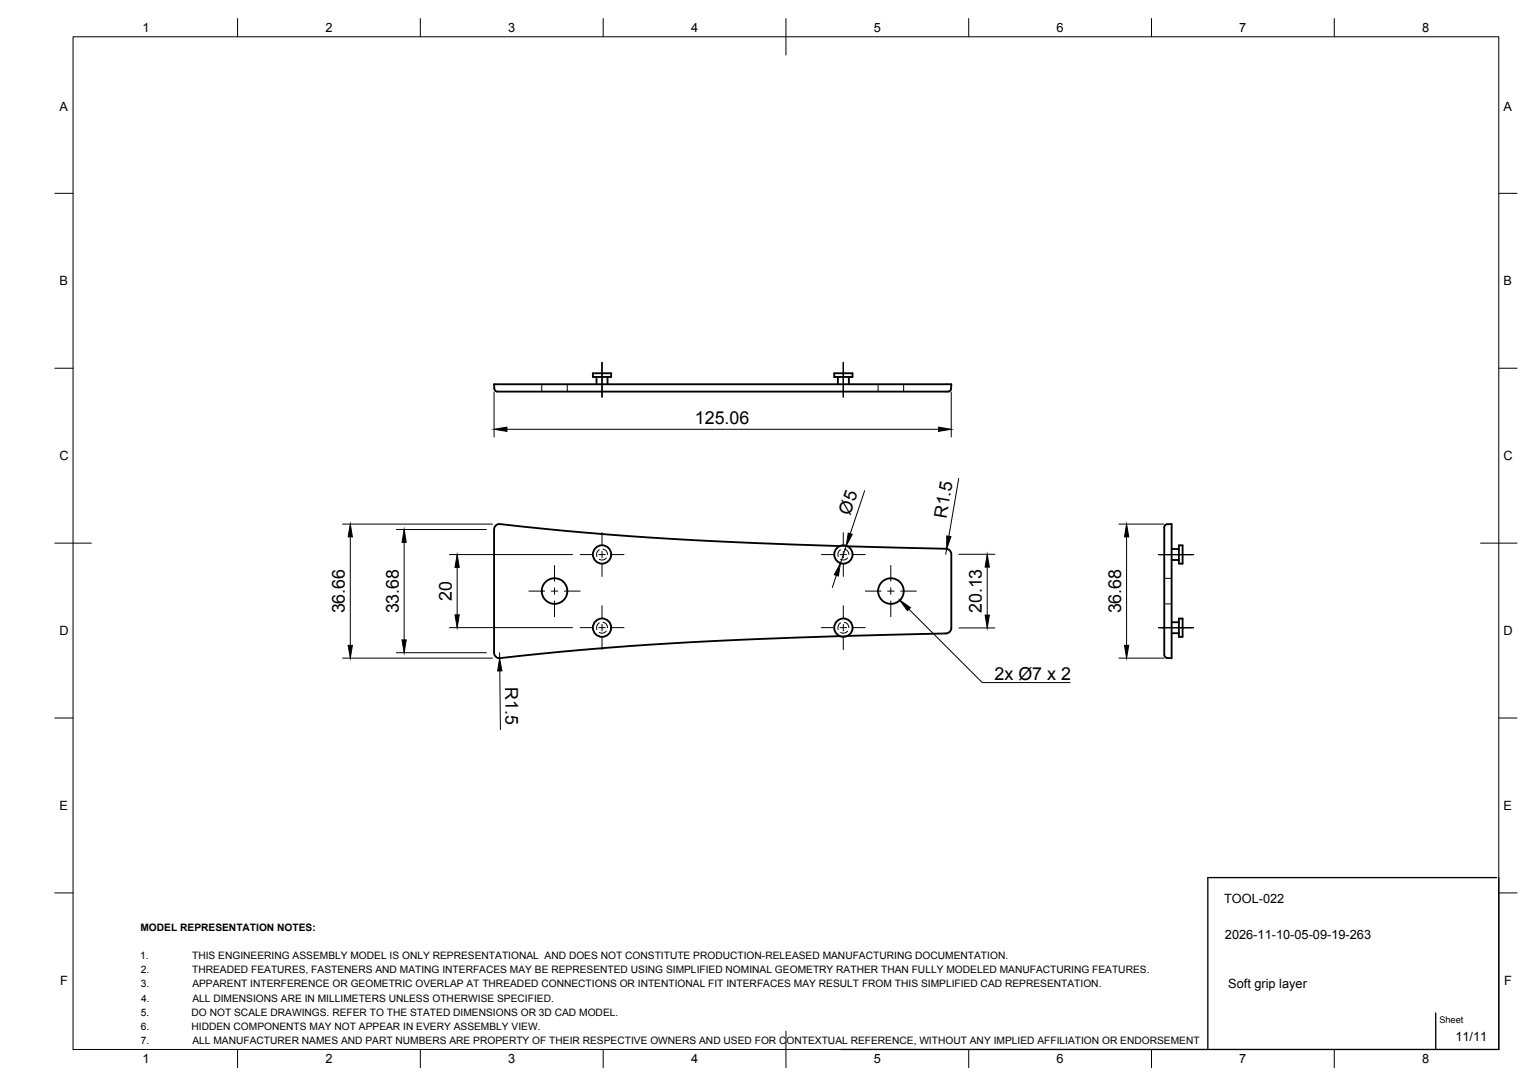
ISO-10303-21;
HEADER;
/* Generated by software containing ST-Developer
 * from STEP Tools, Inc. (www.steptools.com) 
 */

FILE_DESCRIPTION(
/* description */ (''),
/* implementation_level */ '2;1');

FILE_NAME(
/* name */ 'Soft grip layer.step',
/* time_stamp */ '2026-11-10T08:27:36-08:00',
/* author */ (''),
/* organization */ (''),
/* preprocessor_version */ 'ST-DEVELOPER v20.2',
/* originating_system */ 'Autodesk Translation Framework v15.17.0.0',
/* authorisation */ '');

FILE_SCHEMA (('AUTOMOTIVE_DESIGN { 1 0 10303 214 3 1 1 }'));
ENDSEC;

DATA;
#10=MECHANICAL_DESIGN_GEOMETRIC_PRESENTATION_REPRESENTATION('',(#572),#19090);
#156=B_SPLINE_SURFACE_WITH_KNOTS('',3,3,((#13418,#13419,#13420,#13421,#13422),
(#13423,#13424,#13425,#13426,#13427),(#13428,#13429,#13430,#13431,#13432),
(#13433,#13434,#13435,#13436,#13437),(#13438,#13439,#13440,#13441,#13442)),
 .UNSPECIFIED.,.F.,.F.,.F.,(4,1,4),(4,1,4),(0.,0.571428571428571,1.),(0.,
0.0505788685273923,0.118017359897249),.UNSPECIFIED.);
#157=B_SPLINE_SURFACE_WITH_KNOTS('',3,3,((#13465,#13466,#13467,#13468,#13469),
(#13470,#13471,#13472,#13473,#13474),(#13475,#13476,#13477,#13478,#13479),
(#13480,#13481,#13482,#13483,#13484),(#13485,#13486,#13487,#13488,#13489)),
 .UNSPECIFIED.,.F.,.F.,.F.,(4,1,4),(4,1,4),(0.,0.571428571428571,1.),(0.,
0.0505788685278266,0.118017359898262),.UNSPECIFIED.);
#158=B_SPLINE_SURFACE_WITH_KNOTS('',3,3,((#13503,#13504,#13505,#13506,#13507),
(#13508,#13509,#13510,#13511,#13512),(#13513,#13514,#13515,#13516,#13517),
(#13518,#13519,#13520,#13521,#13522),(#13523,#13524,#13525,#13526,#13527)),
 .UNSPECIFIED.,.F.,.F.,.F.,(4,1,4),(4,1,4),(0.,0.571428571428571,1.),(0.,
5.23288834931112,12.2100728150593),.UNSPECIFIED.);
#159=B_SPLINE_SURFACE_WITH_KNOTS('',3,3,((#13541,#13542,#13543,#13544,#13545),
(#13546,#13547,#13548,#13549,#13550),(#13551,#13552,#13553,#13554,#13555),
(#13556,#13557,#13558,#13559,#13560),(#13561,#13562,#13563,#13564,#13565)),
 .UNSPECIFIED.,.F.,.F.,.F.,(4,1,4),(4,1,4),(0.,0.571428571428571,1.),(1.97133828064127E-11,
0.0463413823988794,0.108129892237767),.UNSPECIFIED.);
#160=B_SPLINE_SURFACE_WITH_KNOTS('',3,3,((#13585,#13586,#13587,#13588,#13589),
(#13590,#13591,#13592,#13593,#13594),(#13595,#13596,#13597,#13598,#13599),
(#13600,#13601,#13602,#13603,#13604),(#13605,#13606,#13607,#13608,#13609)),
 .UNSPECIFIED.,.F.,.F.,.F.,(4,1,4),(4,1,4),(0.,0.571428571428571,1.),(0.,
0.0463413823743492,0.108129892206815),.UNSPECIFIED.);
#161=B_SPLINE_SURFACE_WITH_KNOTS('',3,3,((#13623,#13624,#13625,#13626,#13627),
(#13628,#13629,#13630,#13631,#13632),(#13633,#13634,#13635,#13636,#13637),
(#13638,#13639,#13640,#13641,#13642),(#13643,#13644,#13645,#13646,#13647)),
 .UNSPECIFIED.,.F.,.F.,.F.,(4,1,4),(4,1,4),(0.,0.571428571428571,1.),(6.51086303075479E-13,
6.97718480957529,12.2100734167563),.UNSPECIFIED.);
#162=B_SPLINE_SURFACE_WITH_KNOTS('',3,3,((#13670,#13671,#13672,#13673),
(#13674,#13675,#13676,#13677),(#13678,#13679,#13680,#13681),(#13682,#13683,
#13684,#13685),(#13686,#13687,#13688,#13689)),.UNSPECIFIED.,.F.,.F.,.F.,
(4,1,4),(4,4),(0.,0.571428571428571,1.),(-0.00308447593286339,0.124708996845866),
 .UNSPECIFIED.);
#163=B_SPLINE_SURFACE_WITH_KNOTS('',3,3,((#13723,#13724,#13725,#13726),
(#13727,#13728,#13729,#13730),(#13731,#13732,#13733,#13734),(#13735,#13736,
#13737,#13738)),.UNSPECIFIED.,.F.,.F.,.F.,(4,4),(4,4),(0.0116899650356219,
0.986620910196183),(0.,0.621418053543664),.UNSPECIFIED.);
#164=B_SPLINE_SURFACE_WITH_KNOTS('',3,3,((#13748,#13749,#13750,#13751),
(#13752,#13753,#13754,#13755),(#13756,#13757,#13758,#13759),(#13760,#13761,
#13762,#13763),(#13764,#13765,#13766,#13767),(#13768,#13769,#13770,#13771)),
 .UNSPECIFIED.,.F.,.F.,.F.,(4,1,1,4),(4,4),(0.,0.285714285714286,0.571428571428571,
1.),(-0.00421817271916687,0.124025126494243),.UNSPECIFIED.);
#165=B_SPLINE_SURFACE_WITH_KNOTS('',3,3,((#13819,#13820,#13821,#13822),
(#13823,#13824,#13825,#13826),(#13827,#13828,#13829,#13830),(#13831,#13832,
#13833,#13834),(#13835,#13836,#13837,#13838)),.UNSPECIFIED.,.F.,.F.,.F.,
(4,1,4),(4,4),(0.,0.571428571428571,1.),(-0.00306862226109154,0.124708996851356),
 .UNSPECIFIED.);
#166=B_SPLINE_SURFACE_WITH_KNOTS('',3,3,((#13872,#13873,#13874,#13875),
(#13876,#13877,#13878,#13879),(#13880,#13881,#13882,#13883),(#13884,#13885,
#13886,#13887),(#13888,#13889,#13890,#13891),(#13892,#13893,#13894,#13895)),
 .UNSPECIFIED.,.F.,.F.,.F.,(4,1,1,4),(4,4),(0.,0.285714285714286,0.571428571428571,
1.),(-0.00430078538920315,0.12402512649425),.UNSPECIFIED.);
#167=B_SPLINE_SURFACE_WITH_KNOTS('',3,3,((#13940,#13941,#13942,#13943),
(#13944,#13945,#13946,#13947),(#13948,#13949,#13950,#13951),(#13952,#13953,
#13954,#13955)),.UNSPECIFIED.,.F.,.F.,.F.,(4,4),(4,4),(0.0133790898038168,
0.988310034964378),(0.,0.621418053491537),.UNSPECIFIED.);
#364=B_SPLINE_CURVE_WITH_KNOTS('',3,(#13447,#13448,#13449,#13450,#13451),
 .UNSPECIFIED.,.F.,.F.,(4,1,4),(-0.118017359897249,-0.0505788685273923,
0.),.UNSPECIFIED.);
#365=B_SPLINE_CURVE_WITH_KNOTS('',3,(#13454,#13455,#13456,#13457,#13458),
 .UNSPECIFIED.,.F.,.F.,(4,1,4),(0.,0.0505788685273923,0.118017359897249),
 .UNSPECIFIED.);
#366=B_SPLINE_CURVE_WITH_KNOTS('',3,(#13493,#13494,#13495,#13496,#13497),
 .UNSPECIFIED.,.F.,.F.,(4,1,4),(-0.118017359898262,-0.0505788685278266,
0.),.UNSPECIFIED.);
#367=B_SPLINE_CURVE_WITH_KNOTS('',3,(#13498,#13499,#13500,#13501,#13502),
 .UNSPECIFIED.,.F.,.F.,(4,1,4),(0.,0.0505788685278266,0.118017359898262),
 .UNSPECIFIED.);
#368=B_SPLINE_CURVE_WITH_KNOTS('',3,(#13531,#13532,#13533,#13534,#13535),
 .UNSPECIFIED.,.F.,.F.,(4,1,4),(-12.2100728150593,-5.23288834931112,0.),
 .UNSPECIFIED.);
#369=B_SPLINE_CURVE_WITH_KNOTS('',3,(#13536,#13537,#13538,#13539,#13540),
 .UNSPECIFIED.,.F.,.F.,(4,1,4),(0.,5.23288834931112,12.2100728150593),
 .UNSPECIFIED.);
#370=B_SPLINE_CURVE_WITH_KNOTS('',3,(#13569,#13570,#13571,#13572,#13573),
 .UNSPECIFIED.,.F.,.F.,(4,1,4),(-0.108129892237767,-0.0463413823988794,
-1.97133828064127E-11),.UNSPECIFIED.);
#371=B_SPLINE_CURVE_WITH_KNOTS('',3,(#13574,#13575,#13576,#13577,#13578),
 .UNSPECIFIED.,.F.,.F.,(4,1,4),(1.97133828064127E-11,0.0463413823988794,
0.108129892237767),.UNSPECIFIED.);
#372=B_SPLINE_CURVE_WITH_KNOTS('',3,(#13613,#13614,#13615,#13616,#13617),
 .UNSPECIFIED.,.F.,.F.,(4,1,4),(-0.108129892206815,-0.0463413823743492,
0.),.UNSPECIFIED.);
#373=B_SPLINE_CURVE_WITH_KNOTS('',3,(#13618,#13619,#13620,#13621,#13622),
 .UNSPECIFIED.,.F.,.F.,(4,1,4),(0.,0.0463413823743492,0.108129892206815),
 .UNSPECIFIED.);
#374=B_SPLINE_CURVE_WITH_KNOTS('',3,(#13648,#13649,#13650,#13651,#13652),
 .UNSPECIFIED.,.F.,.F.,(4,1,4),(-12.2100734167563,-6.97718480957529,-6.51086303075479E-13),
 .UNSPECIFIED.);
#375=B_SPLINE_CURVE_WITH_KNOTS('',3,(#13653,#13654,#13655,#13656,#13657),
 .UNSPECIFIED.,.F.,.F.,(4,1,4),(6.51086303075479E-13,6.97718480957529,12.2100734167563),
 .UNSPECIFIED.);
#376=B_SPLINE_CURVE_WITH_KNOTS('',3,(#13660,#13661,#13662,#13663),
 .UNSPECIFIED.,.F.,.F.,(4,4),(0.000181689894813921,0.124708996845866),
 .UNSPECIFIED.);
#377=B_SPLINE_CURVE_WITH_KNOTS('',3,(#13666,#13667,#13668,#13669),
 .UNSPECIFIED.,.F.,.F.,(4,4),(-0.124708996851356,-0.000181689894814102),
 .UNSPECIFIED.);
#378=B_SPLINE_CURVE_WITH_KNOTS('',3,(#13691,#13692,#13693,#13694),
 .UNSPECIFIED.,.F.,.F.,(4,4),(-0.124624122980966,-1.27068494615301E-16),
 .UNSPECIFIED.);
#379=B_SPLINE_CURVE_WITH_KNOTS('',3,(#13695,#13696,#13697,#13698,#13699,
#13700,#13701,#13702,#13703,#13704,#13705,#13706,#13707,#13708,#13709,#13710,
#13711,#13712,#13713,#13714,#13715,#13716,#13717,#13718,#13719,#13720,#13721,
#13722),.UNSPECIFIED.,.F.,.F.,(4,3,3,3,3,3,3,3,3,4),(0.,0.0322747504276753,
0.0586406101183928,0.090870813631105,0.0996503787243826,0.117132790114159,
0.149546322800321,0.175583390425035,0.207787925145658,0.232457773984835),
 .UNSPECIFIED.);
#380=B_SPLINE_CURVE_WITH_KNOTS('',3,(#13740,#13741,#13742,#13743),
 .UNSPECIFIED.,.F.,.F.,(4,4),(6.28713621962651E-9,0.124025126494243),
 .UNSPECIFIED.);
#381=B_SPLINE_CURVE_WITH_KNOTS('',3,(#13744,#13745,#13746,#13747),
 .UNSPECIFIED.,.F.,.F.,(4,4),(0.0116899650356219,0.986620910196183),
 .UNSPECIFIED.);
#382=B_SPLINE_CURVE_WITH_KNOTS('',3,(#13773,#13774,#13775,#13776),
 .UNSPECIFIED.,.F.,.F.,(4,4),(-0.12358375933533,0.000944809985246663),
 .UNSPECIFIED.);
#383=B_SPLINE_CURVE_WITH_KNOTS('',3,(#13777,#13778,#13779,#13780,#13781,
#13782,#13783,#13784,#13785,#13786,#13787,#13788,#13789,#13790,#13791,#13792,
#13793,#13794,#13795,#13796,#13797,#13798,#13799,#13800,#13801,#13802,#13803,
#13804,#13805,#13806,#13807,#13808,#13809,#13810),.UNSPECIFIED.,.F.,.F.,
(4,3,3,3,3,3,3,3,3,3,3,4),(0.,0.0322568536241053,0.0586526138523664,0.0909514856947606,
0.108742407475907,0.117151788463556,0.149394351344039,0.175600627102286,
0.181167420983902,0.214570374458228,0.246736309066329,0.253563811229603),
 .UNSPECIFIED.);
#384=B_SPLINE_CURVE_WITH_KNOTS('',3,(#13814,#13815,#13816,#13817),
 .UNSPECIFIED.,.F.,.F.,(4,4),(-0.000944809985246617,0.123583759335329),
 .UNSPECIFIED.);
#385=B_SPLINE_CURVE_WITH_KNOTS('',3,(#13840,#13841,#13842,#13843,#13844,
#13845,#13846,#13847,#13848,#13849,#13850,#13851,#13852,#13853,#13854,#13855,
#13856,#13857,#13858,#13859,#13860,#13861,#13862,#13863,#13864,#13865,#13866,
#13867),.UNSPECIFIED.,.F.,.F.,(4,3,3,3,3,3,3,3,3,4),(0.,0.0322765438584903,
0.0586513922310012,0.0908809480268686,0.099655003871439,0.117150238497558,
0.149564657711791,0.175599638586681,0.20780211537115,0.232458396023953),
 .UNSPECIFIED.);
#386=B_SPLINE_CURVE_WITH_KNOTS('',3,(#13868,#13869,#13870,#13871),
 .UNSPECIFIED.,.F.,.F.,(4,4),(3.30031141304588E-16,0.124624122970512),
 .UNSPECIFIED.);
#387=B_SPLINE_CURVE_WITH_KNOTS('',3,(#13897,#13898,#13899,#13900),
 .UNSPECIFIED.,.F.,.F.,(4,4),(-0.12402512649425,-6.28713634712869E-9),
 .UNSPECIFIED.);
#388=B_SPLINE_CURVE_WITH_KNOTS('',3,(#13901,#13902,#13903,#13904,#13905,
#13906,#13907,#13908,#13909,#13910,#13911,#13912,#13913,#13914,#13915,#13916,
#13917,#13918,#13919,#13920,#13921,#13922,#13923,#13924,#13925,#13926,#13927,
#13928,#13929,#13930,#13931,#13932,#13933,#13934),.UNSPECIFIED.,.F.,.F.,
(4,3,3,3,3,3,3,3,3,3,3,4),(0.,0.0322666769662355,0.0587055335553437,0.0910029078093924,
0.108768157423115,0.117242626226166,0.149488313345073,0.175692943342501,
0.181189289804584,0.214619150478997,0.24677571115805,0.253566775541772),
 .UNSPECIFIED.);
#389=B_SPLINE_CURVE_WITH_KNOTS('',3,(#13936,#13937,#13938,#13939),
 .UNSPECIFIED.,.F.,.F.,(4,4),(0.0133790898038168,0.988310034964378),
 .UNSPECIFIED.);
#552=SHAPE_REPRESENTATION_RELATIONSHIP('SRR','None',#19143,#562);
#562=ADVANCED_BREP_SHAPE_REPRESENTATION('',(#582),#19086);
#572=STYLED_ITEM('',(#19204),#582);
#582=MANIFOLD_SOLID_BREP('Body1',#6826);
#635=FACE_BOUND('',#1503,.T.);
#636=FACE_BOUND('',#1507,.T.);
#637=FACE_BOUND('',#1511,.T.);
#638=FACE_BOUND('',#1515,.T.);
#639=FACE_BOUND('',#1535,.T.);
#640=FACE_BOUND('',#1536,.T.);
#641=FACE_BOUND('',#1541,.T.);
#642=FACE_BOUND('',#1542,.T.);
#643=FACE_BOUND('',#1543,.T.);
#644=FACE_BOUND('',#1544,.T.);
#645=FACE_BOUND('',#1545,.T.);
#646=FACE_BOUND('',#1546,.T.);
#781=PLANE('',#7258);
#782=PLANE('',#7263);
#783=PLANE('',#7264);
#784=PLANE('',#7269);
#785=PLANE('',#7270);
#786=PLANE('',#7275);
#787=PLANE('',#7276);
#788=PLANE('',#7281);
#789=PLANE('',#7300);
#790=PLANE('',#7301);
#791=PLANE('',#7302);
#792=PLANE('',#7303);
#1063=FACE_OUTER_BOUND('',#1500,.T.);
#1064=FACE_OUTER_BOUND('',#1501,.T.);
#1065=FACE_OUTER_BOUND('',#1502,.T.);
#1066=FACE_OUTER_BOUND('',#1504,.T.);
#1067=FACE_OUTER_BOUND('',#1505,.T.);
#1068=FACE_OUTER_BOUND('',#1506,.T.);
#1069=FACE_OUTER_BOUND('',#1508,.T.);
#1070=FACE_OUTER_BOUND('',#1509,.T.);
#1071=FACE_OUTER_BOUND('',#1510,.T.);
#1072=FACE_OUTER_BOUND('',#1512,.T.);
#1073=FACE_OUTER_BOUND('',#1513,.T.);
#1074=FACE_OUTER_BOUND('',#1514,.T.);
#1075=FACE_OUTER_BOUND('',#1516,.T.);
#1076=FACE_OUTER_BOUND('',#1517,.T.);
#1077=FACE_OUTER_BOUND('',#1518,.T.);
#1078=FACE_OUTER_BOUND('',#1519,.T.);
#1079=FACE_OUTER_BOUND('',#1520,.T.);
#1080=FACE_OUTER_BOUND('',#1521,.T.);
#1081=FACE_OUTER_BOUND('',#1522,.T.);
#1082=FACE_OUTER_BOUND('',#1523,.T.);
#1083=FACE_OUTER_BOUND('',#1524,.T.);
#1084=FACE_OUTER_BOUND('',#1525,.T.);
#1085=FACE_OUTER_BOUND('',#1526,.T.);
#1086=FACE_OUTER_BOUND('',#1527,.T.);
#1087=FACE_OUTER_BOUND('',#1528,.T.);
#1088=FACE_OUTER_BOUND('',#1529,.T.);
#1089=FACE_OUTER_BOUND('',#1530,.T.);
#1090=FACE_OUTER_BOUND('',#1531,.T.);
#1091=FACE_OUTER_BOUND('',#1532,.T.);
#1092=FACE_OUTER_BOUND('',#1533,.T.);
#1093=FACE_OUTER_BOUND('',#1534,.T.);
#1094=FACE_OUTER_BOUND('',#1537,.T.);
#1095=FACE_OUTER_BOUND('',#1538,.T.);
#1096=FACE_OUTER_BOUND('',#1539,.T.);
#1097=FACE_OUTER_BOUND('',#1540,.T.);
#1098=FACE_OUTER_BOUND('',#1547,.T.);
#1500=EDGE_LOOP('',(#5597,#5598,#5599,#5600));
#1501=EDGE_LOOP('',(#5601,#5602,#5603,#5604));
#1502=EDGE_LOOP('',(#5605));
#1503=EDGE_LOOP('',(#5606));
#1504=EDGE_LOOP('',(#5607,#5608,#5609,#5610));
#1505=EDGE_LOOP('',(#5611));
#1506=EDGE_LOOP('',(#5612));
#1507=EDGE_LOOP('',(#5613));
#1508=EDGE_LOOP('',(#5614,#5615,#5616,#5617));
#1509=EDGE_LOOP('',(#5618));
#1510=EDGE_LOOP('',(#5619));
#1511=EDGE_LOOP('',(#5620));
#1512=EDGE_LOOP('',(#5621,#5622,#5623,#5624));
#1513=EDGE_LOOP('',(#5625));
#1514=EDGE_LOOP('',(#5626));
#1515=EDGE_LOOP('',(#5627));
#1516=EDGE_LOOP('',(#5628,#5629,#5630,#5631));
#1517=EDGE_LOOP('',(#5632));
#1518=EDGE_LOOP('',(#5633,#5634,#5635,#5636));
#1519=EDGE_LOOP('',(#5637,#5638,#5639,#5640));
#1520=EDGE_LOOP('',(#5641,#5642,#5643,#5644));
#1521=EDGE_LOOP('',(#5645,#5646,#5647,#5648));
#1522=EDGE_LOOP('',(#5649,#5650,#5651,#5652));
#1523=EDGE_LOOP('',(#5653,#5654,#5655,#5656));
#1524=EDGE_LOOP('',(#5657,#5658,#5659,#5660));
#1525=EDGE_LOOP('',(#5661,#5662,#5663,#5664));
#1526=EDGE_LOOP('',(#5665,#5666,#5667,#5668));
#1527=EDGE_LOOP('',(#5669,#5670,#5671,#5672));
#1528=EDGE_LOOP('',(#5673,#5674,#5675,#5676));
#1529=EDGE_LOOP('',(#5677,#5678,#5679,#5680));
#1530=EDGE_LOOP('',(#5681,#5682,#5683,#5684));
#1531=EDGE_LOOP('',(#5685,#5686,#5687,#5688));
#1532=EDGE_LOOP('',(#5689,#5690,#5691,#5692));
#1533=EDGE_LOOP('',(#5693,#5694,#5695,#5696));
#1534=EDGE_LOOP('',(#5697,#5698,#5699,#5700,#5701,#5702,#5703,#5704));
#1535=EDGE_LOOP('',(#5705));
#1536=EDGE_LOOP('',(#5706));
#1537=EDGE_LOOP('',(#5707,#5708,#5709,#5710));
#1538=EDGE_LOOP('',(#5711,#5712,#5713,#5714));
#1539=EDGE_LOOP('',(#5715,#5716,#5717,#5718));
#1540=EDGE_LOOP('',(#5719,#5720,#5721,#5722,#5723,#5724,#5725,#5726));
#1541=EDGE_LOOP('',(#5727));
#1542=EDGE_LOOP('',(#5728));
#1543=EDGE_LOOP('',(#5729));
#1544=EDGE_LOOP('',(#5730));
#1545=EDGE_LOOP('',(#5731));
#1546=EDGE_LOOP('',(#5732));
#1547=EDGE_LOOP('',(#5733,#5734,#5735,#5736));
#1979=LINE('',#13354,#2428);
#1980=LINE('',#13360,#2429);
#1981=LINE('',#13370,#2430);
#1982=LINE('',#13380,#2431);
#1983=LINE('',#13390,#2432);
#1984=LINE('',#13400,#2433);
#1985=LINE('',#13404,#2434);
#1986=LINE('',#13408,#2435);
#1987=LINE('',#13412,#2436);
#1988=LINE('',#13416,#2437);
#1989=LINE('',#13463,#2438);
#1990=LINE('',#13464,#2439);
#1991=LINE('',#13583,#2440);
#1992=LINE('',#13584,#2441);
#1993=LINE('',#13665,#2442);
#1994=LINE('',#13818,#2443);
#2428=VECTOR('',#8386,0.35);
#2429=VECTOR('',#8393,0.35);
#2430=VECTOR('',#8406,0.25);
#2431=VECTOR('',#8419,0.25);
#2432=VECTOR('',#8432,0.25);
#2433=VECTOR('',#8445,0.25);
#2434=VECTOR('',#8450,0.15);
#2435=VECTOR('',#8455,0.15);
#2436=VECTOR('',#8460,0.15);
#2437=VECTOR('',#8465,0.15);
#2438=VECTOR('',#8476,1.);
#2439=VECTOR('',#8477,1.);
#2440=VECTOR('',#8488,1.);
#2441=VECTOR('',#8489,1.);
#2442=VECTOR('',#8494,1.);
#2443=VECTOR('',#8499,1.);
#2670=CIRCLE('',#7253,0.35);
#2671=CIRCLE('',#7254,0.35);
#2672=CIRCLE('',#7256,0.35);
#2673=CIRCLE('',#7257,0.35);
#2674=CIRCLE('',#7259,0.25);
#2675=CIRCLE('',#7260,0.15);
#2676=CIRCLE('',#7262,0.25);
#2677=CIRCLE('',#7265,0.25);
#2678=CIRCLE('',#7266,0.15);
#2679=CIRCLE('',#7268,0.25);
#2680=CIRCLE('',#7271,0.25);
#2681=CIRCLE('',#7272,0.15);
#2682=CIRCLE('',#7274,0.25);
#2683=CIRCLE('',#7277,0.25);
#2684=CIRCLE('',#7278,0.15);
#2685=CIRCLE('',#7280,0.25);
#2686=CIRCLE('',#7283,0.15);
#2687=CIRCLE('',#7285,0.15);
#2688=CIRCLE('',#7287,0.15);
#2689=CIRCLE('',#7289,0.15);
#2690=CIRCLE('',#7290,0.0800000000000001);
#2691=CIRCLE('',#7291,0.0800000000000001);
#2692=CIRCLE('',#7293,0.0800000000000001);
#2693=CIRCLE('',#7294,0.0800000000000001);
#2694=CIRCLE('',#7295,0.0800000000000001);
#2695=CIRCLE('',#7296,0.0800000000000003);
#2696=CIRCLE('',#7298,0.0800000000000001);
#2697=CIRCLE('',#7299,0.0800000000000003);
#3120=VERTEX_POINT('',#13351);
#3121=VERTEX_POINT('',#13353);
#3122=VERTEX_POINT('',#13357);
#3123=VERTEX_POINT('',#13359);
#3124=VERTEX_POINT('',#13363);
#3125=VERTEX_POINT('',#13365);
#3126=VERTEX_POINT('',#13368);
#3127=VERTEX_POINT('',#13373);
#3128=VERTEX_POINT('',#13375);
#3129=VERTEX_POINT('',#13378);
#3130=VERTEX_POINT('',#13383);
#3131=VERTEX_POINT('',#13385);
#3132=VERTEX_POINT('',#13388);
#3133=VERTEX_POINT('',#13393);
#3134=VERTEX_POINT('',#13395);
#3135=VERTEX_POINT('',#13398);
#3136=VERTEX_POINT('',#13403);
#3137=VERTEX_POINT('',#13407);
#3138=VERTEX_POINT('',#13411);
#3139=VERTEX_POINT('',#13415);
#3140=VERTEX_POINT('',#13443);
#3141=VERTEX_POINT('',#13444);
#3142=VERTEX_POINT('',#13446);
#3143=VERTEX_POINT('',#13452);
#3144=VERTEX_POINT('',#13460);
#3145=VERTEX_POINT('',#13461);
#3146=VERTEX_POINT('',#13490);
#3147=VERTEX_POINT('',#13491);
#3148=VERTEX_POINT('',#13528);
#3149=VERTEX_POINT('',#13529);
#3150=VERTEX_POINT('',#13566);
#3151=VERTEX_POINT('',#13567);
#3152=VERTEX_POINT('',#13580);
#3153=VERTEX_POINT('',#13581);
#3154=VERTEX_POINT('',#13610);
#3155=VERTEX_POINT('',#13611);
#3156=VERTEX_POINT('',#13659);
#3157=VERTEX_POINT('',#13664);
#3158=VERTEX_POINT('',#13690);
#3159=VERTEX_POINT('',#13739);
#3160=VERTEX_POINT('',#13772);
#3161=VERTEX_POINT('',#13813);
#3162=VERTEX_POINT('',#13839);
#3163=VERTEX_POINT('',#13896);
#3983=EDGE_CURVE('',#3120,#3120,#2670,.T.);
#3984=EDGE_CURVE('',#3120,#3121,#1979,.T.);
#3985=EDGE_CURVE('',#3121,#3121,#2671,.T.);
#3986=EDGE_CURVE('',#3122,#3122,#2672,.T.);
#3987=EDGE_CURVE('',#3122,#3123,#1980,.T.);
#3988=EDGE_CURVE('',#3123,#3123,#2673,.T.);
#3989=EDGE_CURVE('',#3124,#3124,#2674,.T.);
#3990=EDGE_CURVE('',#3125,#3125,#2675,.T.);
#3991=EDGE_CURVE('',#3126,#3126,#2676,.T.);
#3992=EDGE_CURVE('',#3126,#3124,#1981,.T.);
#3993=EDGE_CURVE('',#3127,#3127,#2677,.T.);
#3994=EDGE_CURVE('',#3128,#3128,#2678,.T.);
#3995=EDGE_CURVE('',#3129,#3129,#2679,.T.);
#3996=EDGE_CURVE('',#3129,#3127,#1982,.T.);
#3997=EDGE_CURVE('',#3130,#3130,#2680,.T.);
#3998=EDGE_CURVE('',#3131,#3131,#2681,.T.);
#3999=EDGE_CURVE('',#3132,#3132,#2682,.T.);
#4000=EDGE_CURVE('',#3132,#3130,#1983,.T.);
#4001=EDGE_CURVE('',#3133,#3133,#2683,.T.);
#4002=EDGE_CURVE('',#3134,#3134,#2684,.T.);
#4003=EDGE_CURVE('',#3135,#3135,#2685,.T.);
#4004=EDGE_CURVE('',#3135,#3133,#1984,.T.);
#4005=EDGE_CURVE('',#3125,#3136,#1985,.T.);
#4006=EDGE_CURVE('',#3136,#3136,#2686,.T.);
#4007=EDGE_CURVE('',#3128,#3137,#1986,.T.);
#4008=EDGE_CURVE('',#3137,#3137,#2687,.T.);
#4009=EDGE_CURVE('',#3131,#3138,#1987,.T.);
#4010=EDGE_CURVE('',#3138,#3138,#2688,.T.);
#4011=EDGE_CURVE('',#3134,#3139,#1988,.T.);
#4012=EDGE_CURVE('',#3139,#3139,#2689,.T.);
#4013=EDGE_CURVE('',#3140,#3141,#2690,.T.);
#4014=EDGE_CURVE('',#3141,#3142,#364,.T.);
#4015=EDGE_CURVE('',#3142,#3143,#2691,.T.);
#4016=EDGE_CURVE('',#3143,#3140,#365,.T.);
#4017=EDGE_CURVE('',#3144,#3145,#2692,.T.);
#4018=EDGE_CURVE('',#3145,#3141,#1989,.T.);
#4019=EDGE_CURVE('',#3140,#3144,#1990,.T.);
#4020=EDGE_CURVE('',#3146,#3147,#2693,.T.);
#4021=EDGE_CURVE('',#3147,#3145,#366,.T.);
#4022=EDGE_CURVE('',#3144,#3146,#367,.T.);
#4023=EDGE_CURVE('',#3148,#3149,#2694,.T.);
#4024=EDGE_CURVE('',#3149,#3147,#368,.T.);
#4025=EDGE_CURVE('',#3146,#3148,#369,.T.);
#4026=EDGE_CURVE('',#3150,#3151,#2695,.T.);
#4027=EDGE_CURVE('',#3151,#3149,#370,.T.);
#4028=EDGE_CURVE('',#3148,#3150,#371,.T.);
#4029=EDGE_CURVE('',#3152,#3153,#2696,.T.);
#4030=EDGE_CURVE('',#3153,#3151,#1991,.T.);
#4031=EDGE_CURVE('',#3150,#3152,#1992,.T.);
#4032=EDGE_CURVE('',#3154,#3155,#2697,.T.);
#4033=EDGE_CURVE('',#3155,#3153,#372,.T.);
#4034=EDGE_CURVE('',#3152,#3154,#373,.T.);
#4035=EDGE_CURVE('',#3142,#3155,#374,.T.);
#4036=EDGE_CURVE('',#3154,#3143,#375,.T.);
#4037=EDGE_CURVE('',#3156,#3153,#376,.T.);
#4038=EDGE_CURVE('',#3157,#3156,#1993,.T.);
#4039=EDGE_CURVE('',#3151,#3157,#377,.T.);
#4040=EDGE_CURVE('',#3155,#3158,#378,.T.);
#4041=EDGE_CURVE('',#3158,#3156,#379,.T.);
#4042=EDGE_CURVE('',#3159,#3142,#380,.T.);
#4043=EDGE_CURVE('',#3158,#3159,#381,.T.);
#4044=EDGE_CURVE('',#3141,#3160,#382,.T.);
#4045=EDGE_CURVE('',#3160,#3159,#383,.T.);
#4046=EDGE_CURVE('',#3161,#3145,#384,.T.);
#4047=EDGE_CURVE('',#3160,#3161,#1994,.T.);
#4048=EDGE_CURVE('',#3157,#3162,#385,.T.);
#4049=EDGE_CURVE('',#3162,#3149,#386,.T.);
#4050=EDGE_CURVE('',#3147,#3163,#387,.T.);
#4051=EDGE_CURVE('',#3163,#3161,#388,.T.);
#4052=EDGE_CURVE('',#3163,#3162,#389,.T.);
#5597=ORIENTED_EDGE('',*,*,#3983,.F.);
#5598=ORIENTED_EDGE('',*,*,#3984,.T.);
#5599=ORIENTED_EDGE('',*,*,#3985,.F.);
#5600=ORIENTED_EDGE('',*,*,#3984,.F.);
#5601=ORIENTED_EDGE('',*,*,#3986,.F.);
#5602=ORIENTED_EDGE('',*,*,#3987,.T.);
#5603=ORIENTED_EDGE('',*,*,#3988,.F.);
#5604=ORIENTED_EDGE('',*,*,#3987,.F.);
#5605=ORIENTED_EDGE('',*,*,#3989,.T.);
#5606=ORIENTED_EDGE('',*,*,#3990,.T.);
#5607=ORIENTED_EDGE('',*,*,#3991,.F.);
#5608=ORIENTED_EDGE('',*,*,#3992,.T.);
#5609=ORIENTED_EDGE('',*,*,#3989,.F.);
#5610=ORIENTED_EDGE('',*,*,#3992,.F.);
#5611=ORIENTED_EDGE('',*,*,#3991,.T.);
#5612=ORIENTED_EDGE('',*,*,#3993,.T.);
#5613=ORIENTED_EDGE('',*,*,#3994,.T.);
#5614=ORIENTED_EDGE('',*,*,#3995,.F.);
#5615=ORIENTED_EDGE('',*,*,#3996,.T.);
#5616=ORIENTED_EDGE('',*,*,#3993,.F.);
#5617=ORIENTED_EDGE('',*,*,#3996,.F.);
#5618=ORIENTED_EDGE('',*,*,#3995,.T.);
#5619=ORIENTED_EDGE('',*,*,#3997,.T.);
#5620=ORIENTED_EDGE('',*,*,#3998,.T.);
#5621=ORIENTED_EDGE('',*,*,#3999,.F.);
#5622=ORIENTED_EDGE('',*,*,#4000,.T.);
#5623=ORIENTED_EDGE('',*,*,#3997,.F.);
#5624=ORIENTED_EDGE('',*,*,#4000,.F.);
#5625=ORIENTED_EDGE('',*,*,#3999,.T.);
#5626=ORIENTED_EDGE('',*,*,#4001,.T.);
#5627=ORIENTED_EDGE('',*,*,#4002,.T.);
#5628=ORIENTED_EDGE('',*,*,#4003,.F.);
#5629=ORIENTED_EDGE('',*,*,#4004,.T.);
#5630=ORIENTED_EDGE('',*,*,#4001,.F.);
#5631=ORIENTED_EDGE('',*,*,#4004,.F.);
#5632=ORIENTED_EDGE('',*,*,#4003,.T.);
#5633=ORIENTED_EDGE('',*,*,#3990,.F.);
#5634=ORIENTED_EDGE('',*,*,#4005,.T.);
#5635=ORIENTED_EDGE('',*,*,#4006,.F.);
#5636=ORIENTED_EDGE('',*,*,#4005,.F.);
#5637=ORIENTED_EDGE('',*,*,#3994,.F.);
#5638=ORIENTED_EDGE('',*,*,#4007,.T.);
#5639=ORIENTED_EDGE('',*,*,#4008,.F.);
#5640=ORIENTED_EDGE('',*,*,#4007,.F.);
#5641=ORIENTED_EDGE('',*,*,#3998,.F.);
#5642=ORIENTED_EDGE('',*,*,#4009,.T.);
#5643=ORIENTED_EDGE('',*,*,#4010,.F.);
#5644=ORIENTED_EDGE('',*,*,#4009,.F.);
#5645=ORIENTED_EDGE('',*,*,#4002,.F.);
#5646=ORIENTED_EDGE('',*,*,#4011,.T.);
#5647=ORIENTED_EDGE('',*,*,#4012,.F.);
#5648=ORIENTED_EDGE('',*,*,#4011,.F.);
#5649=ORIENTED_EDGE('',*,*,#4013,.T.);
#5650=ORIENTED_EDGE('',*,*,#4014,.T.);
#5651=ORIENTED_EDGE('',*,*,#4015,.T.);
#5652=ORIENTED_EDGE('',*,*,#4016,.T.);
#5653=ORIENTED_EDGE('',*,*,#4017,.T.);
#5654=ORIENTED_EDGE('',*,*,#4018,.T.);
#5655=ORIENTED_EDGE('',*,*,#4013,.F.);
#5656=ORIENTED_EDGE('',*,*,#4019,.T.);
#5657=ORIENTED_EDGE('',*,*,#4020,.T.);
#5658=ORIENTED_EDGE('',*,*,#4021,.T.);
#5659=ORIENTED_EDGE('',*,*,#4017,.F.);
#5660=ORIENTED_EDGE('',*,*,#4022,.T.);
#5661=ORIENTED_EDGE('',*,*,#4023,.T.);
#5662=ORIENTED_EDGE('',*,*,#4024,.T.);
#5663=ORIENTED_EDGE('',*,*,#4020,.F.);
#5664=ORIENTED_EDGE('',*,*,#4025,.T.);
#5665=ORIENTED_EDGE('',*,*,#4026,.T.);
#5666=ORIENTED_EDGE('',*,*,#4027,.T.);
#5667=ORIENTED_EDGE('',*,*,#4023,.F.);
#5668=ORIENTED_EDGE('',*,*,#4028,.T.);
#5669=ORIENTED_EDGE('',*,*,#4029,.T.);
#5670=ORIENTED_EDGE('',*,*,#4030,.T.);
#5671=ORIENTED_EDGE('',*,*,#4026,.F.);
#5672=ORIENTED_EDGE('',*,*,#4031,.T.);
#5673=ORIENTED_EDGE('',*,*,#4032,.T.);
#5674=ORIENTED_EDGE('',*,*,#4033,.T.);
#5675=ORIENTED_EDGE('',*,*,#4029,.F.);
#5676=ORIENTED_EDGE('',*,*,#4034,.T.);
#5677=ORIENTED_EDGE('',*,*,#4015,.F.);
#5678=ORIENTED_EDGE('',*,*,#4035,.T.);
#5679=ORIENTED_EDGE('',*,*,#4032,.F.);
#5680=ORIENTED_EDGE('',*,*,#4036,.T.);
#5681=ORIENTED_EDGE('',*,*,#4030,.F.);
#5682=ORIENTED_EDGE('',*,*,#4037,.F.);
#5683=ORIENTED_EDGE('',*,*,#4038,.F.);
#5684=ORIENTED_EDGE('',*,*,#4039,.F.);
#5685=ORIENTED_EDGE('',*,*,#4033,.F.);
#5686=ORIENTED_EDGE('',*,*,#4040,.T.);
#5687=ORIENTED_EDGE('',*,*,#4041,.T.);
#5688=ORIENTED_EDGE('',*,*,#4037,.T.);
#5689=ORIENTED_EDGE('',*,*,#4035,.F.);
#5690=ORIENTED_EDGE('',*,*,#4042,.F.);
#5691=ORIENTED_EDGE('',*,*,#4043,.F.);
#5692=ORIENTED_EDGE('',*,*,#4040,.F.);
#5693=ORIENTED_EDGE('',*,*,#4014,.F.);
#5694=ORIENTED_EDGE('',*,*,#4044,.T.);
#5695=ORIENTED_EDGE('',*,*,#4045,.T.);
#5696=ORIENTED_EDGE('',*,*,#4042,.T.);
#5697=ORIENTED_EDGE('',*,*,#4016,.F.);
#5698=ORIENTED_EDGE('',*,*,#4036,.F.);
#5699=ORIENTED_EDGE('',*,*,#4034,.F.);
#5700=ORIENTED_EDGE('',*,*,#4031,.F.);
#5701=ORIENTED_EDGE('',*,*,#4028,.F.);
#5702=ORIENTED_EDGE('',*,*,#4025,.F.);
#5703=ORIENTED_EDGE('',*,*,#4022,.F.);
#5704=ORIENTED_EDGE('',*,*,#4019,.F.);
#5705=ORIENTED_EDGE('',*,*,#3983,.T.);
#5706=ORIENTED_EDGE('',*,*,#3986,.T.);
#5707=ORIENTED_EDGE('',*,*,#4018,.F.);
#5708=ORIENTED_EDGE('',*,*,#4046,.F.);
#5709=ORIENTED_EDGE('',*,*,#4047,.F.);
#5710=ORIENTED_EDGE('',*,*,#4044,.F.);
#5711=ORIENTED_EDGE('',*,*,#4027,.F.);
#5712=ORIENTED_EDGE('',*,*,#4039,.T.);
#5713=ORIENTED_EDGE('',*,*,#4048,.T.);
#5714=ORIENTED_EDGE('',*,*,#4049,.T.);
#5715=ORIENTED_EDGE('',*,*,#4021,.F.);
#5716=ORIENTED_EDGE('',*,*,#4050,.T.);
#5717=ORIENTED_EDGE('',*,*,#4051,.T.);
#5718=ORIENTED_EDGE('',*,*,#4046,.T.);
#5719=ORIENTED_EDGE('',*,*,#4045,.F.);
#5720=ORIENTED_EDGE('',*,*,#4047,.T.);
#5721=ORIENTED_EDGE('',*,*,#4051,.F.);
#5722=ORIENTED_EDGE('',*,*,#4052,.T.);
#5723=ORIENTED_EDGE('',*,*,#4048,.F.);
#5724=ORIENTED_EDGE('',*,*,#4038,.T.);
#5725=ORIENTED_EDGE('',*,*,#4041,.F.);
#5726=ORIENTED_EDGE('',*,*,#4043,.T.);
#5727=ORIENTED_EDGE('',*,*,#3985,.T.);
#5728=ORIENTED_EDGE('',*,*,#3988,.T.);
#5729=ORIENTED_EDGE('',*,*,#4006,.T.);
#5730=ORIENTED_EDGE('',*,*,#4008,.T.);
#5731=ORIENTED_EDGE('',*,*,#4010,.T.);
#5732=ORIENTED_EDGE('',*,*,#4012,.T.);
#5733=ORIENTED_EDGE('',*,*,#4024,.F.);
#5734=ORIENTED_EDGE('',*,*,#4049,.F.);
#5735=ORIENTED_EDGE('',*,*,#4052,.F.);
#5736=ORIENTED_EDGE('',*,*,#4050,.F.);
#6343=CYLINDRICAL_SURFACE('',#7252,0.35);
#6344=CYLINDRICAL_SURFACE('',#7255,0.35);
#6345=CYLINDRICAL_SURFACE('',#7261,0.25);
#6346=CYLINDRICAL_SURFACE('',#7267,0.25);
#6347=CYLINDRICAL_SURFACE('',#7273,0.25);
#6348=CYLINDRICAL_SURFACE('',#7279,0.25);
#6349=CYLINDRICAL_SURFACE('',#7282,0.15);
#6350=CYLINDRICAL_SURFACE('',#7284,0.15);
#6351=CYLINDRICAL_SURFACE('',#7286,0.15);
#6352=CYLINDRICAL_SURFACE('',#7288,0.15);
#6353=CYLINDRICAL_SURFACE('',#7292,0.08);
#6354=CYLINDRICAL_SURFACE('',#7297,0.08);
#6682=ADVANCED_FACE('',(#1063),#6343,.F.);
#6683=ADVANCED_FACE('',(#1064),#6344,.F.);
#6684=ADVANCED_FACE('',(#1065,#635),#781,.T.);
#6685=ADVANCED_FACE('',(#1066),#6345,.T.);
#6686=ADVANCED_FACE('',(#1067),#782,.F.);
#6687=ADVANCED_FACE('',(#1068,#636),#783,.T.);
#6688=ADVANCED_FACE('',(#1069),#6346,.T.);
#6689=ADVANCED_FACE('',(#1070),#784,.F.);
#6690=ADVANCED_FACE('',(#1071,#637),#785,.T.);
#6691=ADVANCED_FACE('',(#1072),#6347,.T.);
#6692=ADVANCED_FACE('',(#1073),#786,.F.);
#6693=ADVANCED_FACE('',(#1074,#638),#787,.T.);
#6694=ADVANCED_FACE('',(#1075),#6348,.T.);
#6695=ADVANCED_FACE('',(#1076),#788,.F.);
#6696=ADVANCED_FACE('',(#1077),#6349,.T.);
#6697=ADVANCED_FACE('',(#1078),#6350,.T.);
#6698=ADVANCED_FACE('',(#1079),#6351,.T.);
#6699=ADVANCED_FACE('',(#1080),#6352,.T.);
#6700=ADVANCED_FACE('',(#1081),#156,.F.);
#6701=ADVANCED_FACE('',(#1082),#6353,.T.);
#6702=ADVANCED_FACE('',(#1083),#157,.F.);
#6703=ADVANCED_FACE('',(#1084),#158,.F.);
#6704=ADVANCED_FACE('',(#1085),#159,.F.);
#6705=ADVANCED_FACE('',(#1086),#6354,.T.);
#6706=ADVANCED_FACE('',(#1087),#160,.F.);
#6707=ADVANCED_FACE('',(#1088),#161,.F.);
#6708=ADVANCED_FACE('',(#1089),#789,.F.);
#6709=ADVANCED_FACE('',(#1090),#162,.F.);
#6710=ADVANCED_FACE('',(#1091),#163,.F.);
#6711=ADVANCED_FACE('',(#1092),#164,.F.);
#6712=ADVANCED_FACE('',(#1093,#639,#640),#790,.T.);
#6713=ADVANCED_FACE('',(#1094),#791,.F.);
#6714=ADVANCED_FACE('',(#1095),#165,.F.);
#6715=ADVANCED_FACE('',(#1096),#166,.F.);
#6716=ADVANCED_FACE('',(#1097,#641,#642,#643,#644,#645,#646),#792,.F.);
#6717=ADVANCED_FACE('',(#1098),#167,.F.);
#6826=CLOSED_SHELL('',(#6682,#6683,#6684,#6685,#6686,#6687,#6688,#6689,
#6690,#6691,#6692,#6693,#6694,#6695,#6696,#6697,#6698,#6699,#6700,#6701,
#6702,#6703,#6704,#6705,#6706,#6707,#6708,#6709,#6710,#6711,#6712,#6713,
#6714,#6715,#6716,#6717));
#7251=AXIS2_PLACEMENT_3D('',#13349,#8380,#8381);
#7252=AXIS2_PLACEMENT_3D('',#13350,#8382,#8383);
#7253=AXIS2_PLACEMENT_3D('',#13352,#8384,#8385);
#7254=AXIS2_PLACEMENT_3D('',#13355,#8387,#8388);
#7255=AXIS2_PLACEMENT_3D('',#13356,#8389,#8390);
#7256=AXIS2_PLACEMENT_3D('',#13358,#8391,#8392);
#7257=AXIS2_PLACEMENT_3D('',#13361,#8394,#8395);
#7258=AXIS2_PLACEMENT_3D('',#13362,#8396,#8397);
#7259=AXIS2_PLACEMENT_3D('',#13364,#8398,#8399);
#7260=AXIS2_PLACEMENT_3D('',#13366,#8400,#8401);
#7261=AXIS2_PLACEMENT_3D('',#13367,#8402,#8403);
#7262=AXIS2_PLACEMENT_3D('',#13369,#8404,#8405);
#7263=AXIS2_PLACEMENT_3D('',#13371,#8407,#8408);
#7264=AXIS2_PLACEMENT_3D('',#13372,#8409,#8410);
#7265=AXIS2_PLACEMENT_3D('',#13374,#8411,#8412);
#7266=AXIS2_PLACEMENT_3D('',#13376,#8413,#8414);
#7267=AXIS2_PLACEMENT_3D('',#13377,#8415,#8416);
#7268=AXIS2_PLACEMENT_3D('',#13379,#8417,#8418);
#7269=AXIS2_PLACEMENT_3D('',#13381,#8420,#8421);
#7270=AXIS2_PLACEMENT_3D('',#13382,#8422,#8423);
#7271=AXIS2_PLACEMENT_3D('',#13384,#8424,#8425);
#7272=AXIS2_PLACEMENT_3D('',#13386,#8426,#8427);
#7273=AXIS2_PLACEMENT_3D('',#13387,#8428,#8429);
#7274=AXIS2_PLACEMENT_3D('',#13389,#8430,#8431);
#7275=AXIS2_PLACEMENT_3D('',#13391,#8433,#8434);
#7276=AXIS2_PLACEMENT_3D('',#13392,#8435,#8436);
#7277=AXIS2_PLACEMENT_3D('',#13394,#8437,#8438);
#7278=AXIS2_PLACEMENT_3D('',#13396,#8439,#8440);
#7279=AXIS2_PLACEMENT_3D('',#13397,#8441,#8442);
#7280=AXIS2_PLACEMENT_3D('',#13399,#8443,#8444);
#7281=AXIS2_PLACEMENT_3D('',#13401,#8446,#8447);
#7282=AXIS2_PLACEMENT_3D('',#13402,#8448,#8449);
#7283=AXIS2_PLACEMENT_3D('',#13405,#8451,#8452);
#7284=AXIS2_PLACEMENT_3D('',#13406,#8453,#8454);
#7285=AXIS2_PLACEMENT_3D('',#13409,#8456,#8457);
#7286=AXIS2_PLACEMENT_3D('',#13410,#8458,#8459);
#7287=AXIS2_PLACEMENT_3D('',#13413,#8461,#8462);
#7288=AXIS2_PLACEMENT_3D('',#13414,#8463,#8464);
#7289=AXIS2_PLACEMENT_3D('',#13417,#8466,#8467);
#7290=AXIS2_PLACEMENT_3D('',#13445,#8468,#8469);
#7291=AXIS2_PLACEMENT_3D('',#13453,#8470,#8471);
#7292=AXIS2_PLACEMENT_3D('',#13459,#8472,#8473);
#7293=AXIS2_PLACEMENT_3D('',#13462,#8474,#8475);
#7294=AXIS2_PLACEMENT_3D('',#13492,#8478,#8479);
#7295=AXIS2_PLACEMENT_3D('',#13530,#8480,#8481);
#7296=AXIS2_PLACEMENT_3D('',#13568,#8482,#8483);
#7297=AXIS2_PLACEMENT_3D('',#13579,#8484,#8485);
#7298=AXIS2_PLACEMENT_3D('',#13582,#8486,#8487);
#7299=AXIS2_PLACEMENT_3D('',#13612,#8490,#8491);
#7300=AXIS2_PLACEMENT_3D('',#13658,#8492,#8493);
#7301=AXIS2_PLACEMENT_3D('',#13811,#8495,#8496);
#7302=AXIS2_PLACEMENT_3D('',#13812,#8497,#8498);
#7303=AXIS2_PLACEMENT_3D('',#13935,#8500,#8501);
#8380=DIRECTION('axis',(0.,0.,1.));
#8381=DIRECTION('refdir',(1.,0.,0.));
#8382=DIRECTION('center_axis',(0.,0.,-1.));
#8383=DIRECTION('ref_axis',(1.,0.,0.));
#8384=DIRECTION('center_axis',(-6.04309184969008E-32,-6.38489691472444E-32,
-1.));
#8385=DIRECTION('ref_axis',(1.,0.,0.));
#8386=DIRECTION('',(0.,0.,-1.));
#8387=DIRECTION('center_axis',(1.44549646912992E-31,1.50240180416177E-18,
1.));
#8388=DIRECTION('ref_axis',(1.,0.,0.));
#8389=DIRECTION('center_axis',(0.,0.,-1.));
#8390=DIRECTION('ref_axis',(1.,0.,0.));
#8391=DIRECTION('center_axis',(-6.04309184969008E-32,-6.38489691472444E-32,
-1.));
#8392=DIRECTION('ref_axis',(1.,0.,0.));
#8393=DIRECTION('',(0.,0.,-1.));
#8394=DIRECTION('center_axis',(1.44549646912992E-31,1.50240180416177E-18,
1.));
#8395=DIRECTION('ref_axis',(1.,0.,0.));
#8396=DIRECTION('center_axis',(0.,0.,1.));
#8397=DIRECTION('ref_axis',(1.,0.,0.));
#8398=DIRECTION('center_axis',(0.,0.,1.));
#8399=DIRECTION('ref_axis',(1.,0.,0.));
#8400=DIRECTION('center_axis',(0.,0.,-1.));
#8401=DIRECTION('ref_axis',(1.,0.,0.));
#8402=DIRECTION('center_axis',(0.,0.,-1.));
#8403=DIRECTION('ref_axis',(1.,0.,0.));
#8404=DIRECTION('center_axis',(0.,0.,-1.));
#8405=DIRECTION('ref_axis',(1.,0.,0.));
#8406=DIRECTION('',(0.,0.,1.));
#8407=DIRECTION('center_axis',(0.,0.,1.));
#8408=DIRECTION('ref_axis',(1.,0.,0.));
#8409=DIRECTION('center_axis',(0.,0.,1.));
#8410=DIRECTION('ref_axis',(1.,0.,0.));
#8411=DIRECTION('center_axis',(0.,0.,1.));
#8412=DIRECTION('ref_axis',(1.,0.,0.));
#8413=DIRECTION('center_axis',(0.,0.,-1.));
#8414=DIRECTION('ref_axis',(1.,0.,0.));
#8415=DIRECTION('center_axis',(0.,0.,-1.));
#8416=DIRECTION('ref_axis',(1.,0.,0.));
#8417=DIRECTION('center_axis',(0.,0.,-1.));
#8418=DIRECTION('ref_axis',(1.,0.,0.));
#8419=DIRECTION('',(0.,0.,1.));
#8420=DIRECTION('center_axis',(0.,0.,1.));
#8421=DIRECTION('ref_axis',(1.,0.,0.));
#8422=DIRECTION('center_axis',(0.,0.,1.));
#8423=DIRECTION('ref_axis',(1.,0.,0.));
#8424=DIRECTION('center_axis',(0.,0.,1.));
#8425=DIRECTION('ref_axis',(1.,0.,0.));
#8426=DIRECTION('center_axis',(0.,0.,-1.));
#8427=DIRECTION('ref_axis',(1.,0.,0.));
#8428=DIRECTION('center_axis',(0.,0.,-1.));
#8429=DIRECTION('ref_axis',(1.,0.,0.));
#8430=DIRECTION('center_axis',(0.,0.,-1.));
#8431=DIRECTION('ref_axis',(1.,0.,0.));
#8432=DIRECTION('',(0.,0.,1.));
#8433=DIRECTION('center_axis',(0.,0.,1.));
#8434=DIRECTION('ref_axis',(1.,0.,0.));
#8435=DIRECTION('center_axis',(0.,0.,1.));
#8436=DIRECTION('ref_axis',(1.,0.,0.));
#8437=DIRECTION('center_axis',(0.,0.,1.));
#8438=DIRECTION('ref_axis',(1.,0.,0.));
#8439=DIRECTION('center_axis',(0.,0.,-1.));
#8440=DIRECTION('ref_axis',(1.,0.,0.));
#8441=DIRECTION('center_axis',(0.,0.,-1.));
#8442=DIRECTION('ref_axis',(1.,0.,0.));
#8443=DIRECTION('center_axis',(0.,0.,-1.));
#8444=DIRECTION('ref_axis',(1.,0.,0.));
#8445=DIRECTION('',(0.,0.,1.));
#8446=DIRECTION('center_axis',(0.,0.,1.));
#8447=DIRECTION('ref_axis',(1.,0.,0.));
#8448=DIRECTION('center_axis',(0.,0.,-1.));
#8449=DIRECTION('ref_axis',(1.,0.,0.));
#8450=DIRECTION('',(0.,0.,1.));
#8451=DIRECTION('center_axis',(1.44549646912992E-31,1.50240180416177E-18,
1.));
#8452=DIRECTION('ref_axis',(1.,0.,0.));
#8453=DIRECTION('center_axis',(0.,0.,-1.));
#8454=DIRECTION('ref_axis',(1.,0.,0.));
#8455=DIRECTION('',(0.,0.,1.));
#8456=DIRECTION('center_axis',(1.44549646912992E-31,1.50240180416177E-18,
1.));
#8457=DIRECTION('ref_axis',(1.,0.,0.));
#8458=DIRECTION('center_axis',(0.,0.,-1.));
#8459=DIRECTION('ref_axis',(1.,0.,0.));
#8460=DIRECTION('',(0.,0.,1.));
#8461=DIRECTION('center_axis',(1.44549646912992E-31,1.50240180416177E-18,
1.));
#8462=DIRECTION('ref_axis',(1.,0.,0.));
#8463=DIRECTION('center_axis',(0.,0.,-1.));
#8464=DIRECTION('ref_axis',(1.,0.,0.));
#8465=DIRECTION('',(0.,0.,1.));
#8466=DIRECTION('center_axis',(1.44549646912992E-31,1.50240180416177E-18,
1.));
#8467=DIRECTION('ref_axis',(1.,0.,0.));
#8468=DIRECTION('center_axis',(0.,1.,0.));
#8469=DIRECTION('ref_axis',(0.,0.,1.));
#8470=DIRECTION('center_axis',(0.993165917563083,0.116711011438853,0.));
#8471=DIRECTION('ref_axis',(-0.116587207627638,0.992112394641407,0.0460480120795941));
#8472=DIRECTION('center_axis',(-3.34618268251883E-33,-1.,6.38489691472444E-32));
#8473=DIRECTION('ref_axis',(0.688354575693762,0.,0.72537437101228));
#8474=DIRECTION('center_axis',(0.,1.,0.));
#8475=DIRECTION('ref_axis',(0.,0.,1.));
#8476=DIRECTION('',(3.34618268251883E-33,1.,-6.38489691472444E-32));
#8477=DIRECTION('',(-3.34618268251883E-33,-1.,6.38489691472444E-32));
#8478=DIRECTION('center_axis',(0.993165917563077,-0.116711011438899,0.));
#8479=DIRECTION('ref_axis',(0.,0.,1.));
#8480=DIRECTION('center_axis',(0.999711469489423,-0.0240203615980049,0.));
#8481=DIRECTION('ref_axis',(0.,0.,1.));
#8482=DIRECTION('center_axis',(-3.69655756055634E-12,-1.,2.05200165779092E-26));
#8483=DIRECTION('ref_axis',(5.55111512312576E-15,0.,1.));
#8484=DIRECTION('center_axis',(-3.3461826825185E-33,1.,-6.38489691472444E-32));
#8485=DIRECTION('ref_axis',(-0.688354575693751,0.,0.72537437101229));
#8486=DIRECTION('center_axis',(0.,-1.,0.));
#8487=DIRECTION('ref_axis',(0.,0.,1.));
#8488=DIRECTION('',(3.3461826825185E-33,-1.,6.38489691472444E-32));
#8489=DIRECTION('',(-3.3461826825185E-33,1.,-6.38489691472444E-32));
#8490=DIRECTION('center_axis',(-0.999711469481833,-0.0240203619138888,2.77475672850144E-15));
#8491=DIRECTION('ref_axis',(2.77555756156288E-15,0.,1.));
#8492=DIRECTION('center_axis',(0.998629534754574,0.,-0.0523359562429439));
#8493=DIRECTION('ref_axis',(-0.0523359562429439,0.,-0.998629534754574));
#8494=DIRECTION('',(0.,1.,0.));
#8495=DIRECTION('center_axis',(6.04309184969008E-32,6.38489691472444E-32,
1.));
#8496=DIRECTION('ref_axis',(1.,0.,-6.04309184969008E-32));
#8497=DIRECTION('center_axis',(-0.998629534754574,0.,-0.0523359562429491));
#8498=DIRECTION('ref_axis',(-0.0523359562429491,0.,0.998629534754574));
#8499=DIRECTION('',(0.,-1.,0.));
#8500=DIRECTION('center_axis',(1.44549646912992E-31,1.50240180416177E-18,
1.));
#8501=DIRECTION('ref_axis',(1.,0.,-1.44549646912992E-31));
#13349=CARTESIAN_POINT('',(0.,0.,0.));
#13350=CARTESIAN_POINT('Origin',(2.,0.,1.));
#13351=CARTESIAN_POINT('',(1.65,4.28626379701574E-17,1.1));
#13352=CARTESIAN_POINT('Origin',(2.,0.,1.1));
#13353=CARTESIAN_POINT('',(1.65,4.28626379701574E-17,0.9));
#13354=CARTESIAN_POINT('',(1.65,4.28626379701574E-17,1.));
#13355=CARTESIAN_POINT('Origin',(2.,0.,0.9));
#13356=CARTESIAN_POINT('Origin',(11.2,0.,1.));
#13357=CARTESIAN_POINT('',(10.85,4.28626379701574E-17,1.1));
#13358=CARTESIAN_POINT('Origin',(11.2,0.,1.1));
#13359=CARTESIAN_POINT('',(10.85,4.28626379701574E-17,0.9));
#13360=CARTESIAN_POINT('',(10.85,4.28626379701574E-17,1.));
#13361=CARTESIAN_POINT('Origin',(11.2,0.,0.9));
#13362=CARTESIAN_POINT('Origin',(9.9,1.,0.7));
#13363=CARTESIAN_POINT('',(9.65,1.,0.7));
#13364=CARTESIAN_POINT('Origin',(9.9,1.,0.7));
#13365=CARTESIAN_POINT('',(9.75,1.,0.7));
#13366=CARTESIAN_POINT('Origin',(9.9,1.,0.7));
#13367=CARTESIAN_POINT('Origin',(9.9,1.,0.7));
#13368=CARTESIAN_POINT('',(9.65,1.,0.6));
#13369=CARTESIAN_POINT('Origin',(9.9,1.,0.6));
#13370=CARTESIAN_POINT('',(9.65,1.,0.7));
#13371=CARTESIAN_POINT('Origin',(9.9,1.,0.6));
#13372=CARTESIAN_POINT('Origin',(3.3,-1.,0.7));
#13373=CARTESIAN_POINT('',(3.05,-1.,0.7));
#13374=CARTESIAN_POINT('Origin',(3.3,-1.,0.7));
#13375=CARTESIAN_POINT('',(3.15,-1.,0.7));
#13376=CARTESIAN_POINT('Origin',(3.3,-1.,0.7));
#13377=CARTESIAN_POINT('Origin',(3.3,-1.,0.7));
#13378=CARTESIAN_POINT('',(3.05,-1.,0.6));
#13379=CARTESIAN_POINT('Origin',(3.3,-1.,0.6));
#13380=CARTESIAN_POINT('',(3.05,-1.,0.7));
#13381=CARTESIAN_POINT('Origin',(3.3,-1.,0.6));
#13382=CARTESIAN_POINT('Origin',(3.3,1.,0.7));
#13383=CARTESIAN_POINT('',(3.05,1.,0.7));
#13384=CARTESIAN_POINT('Origin',(3.3,1.,0.7));
#13385=CARTESIAN_POINT('',(3.15,1.,0.7));
#13386=CARTESIAN_POINT('Origin',(3.3,1.,0.7));
#13387=CARTESIAN_POINT('Origin',(3.3,1.,0.7));
#13388=CARTESIAN_POINT('',(3.05,1.,0.6));
#13389=CARTESIAN_POINT('Origin',(3.3,1.,0.6));
#13390=CARTESIAN_POINT('',(3.05,1.,0.7));
#13391=CARTESIAN_POINT('Origin',(3.3,1.,0.6));
#13392=CARTESIAN_POINT('Origin',(9.9,-1.,0.7));
#13393=CARTESIAN_POINT('',(9.65,-1.,0.7));
#13394=CARTESIAN_POINT('Origin',(9.9,-1.,0.7));
#13395=CARTESIAN_POINT('',(9.75,-1.,0.7));
#13396=CARTESIAN_POINT('Origin',(9.9,-1.,0.7));
#13397=CARTESIAN_POINT('Origin',(9.9,-1.,0.7));
#13398=CARTESIAN_POINT('',(9.65,-1.,0.6));
#13399=CARTESIAN_POINT('Origin',(9.9,-1.,0.6));
#13400=CARTESIAN_POINT('',(9.65,-1.,0.7));
#13401=CARTESIAN_POINT('Origin',(9.9,-1.,0.6));
#13402=CARTESIAN_POINT('Origin',(9.9,1.,0.9));
#13403=CARTESIAN_POINT('',(9.75,1.,0.9));
#13404=CARTESIAN_POINT('',(9.75,1.,0.9));
#13405=CARTESIAN_POINT('Origin',(9.9,1.,0.9));
#13406=CARTESIAN_POINT('Origin',(3.3,-1.,0.9));
#13407=CARTESIAN_POINT('',(3.15,-1.,0.9));
#13408=CARTESIAN_POINT('',(3.15,-1.,0.9));
#13409=CARTESIAN_POINT('Origin',(3.3,-1.,0.9));
#13410=CARTESIAN_POINT('Origin',(3.3,1.,0.9));
#13411=CARTESIAN_POINT('',(3.15,1.,0.9));
#13412=CARTESIAN_POINT('',(3.15,1.,0.9));
#13413=CARTESIAN_POINT('Origin',(3.3,1.,0.9));
#13414=CARTESIAN_POINT('Origin',(9.9,-1.,0.9));
#13415=CARTESIAN_POINT('',(9.75,-1.,0.9));
#13416=CARTESIAN_POINT('',(9.75,-1.,0.9));
#13417=CARTESIAN_POINT('Origin',(9.9,-1.,0.9));
#13418=CARTESIAN_POINT('Ctrl Pts',(12.6883460378814,1.74710477827991,1.1));
#13419=CARTESIAN_POINT('Ctrl Pts',(12.7050904406715,1.74907248191433,1.1));
#13420=CARTESIAN_POINT('Ctrl Pts',(12.7459721545883,1.73893278412019,1.1));
#13421=CARTESIAN_POINT('Ctrl Pts',(12.7664342774515,1.70015954799943,1.1));
#13422=CARTESIAN_POINT('Ctrl Pts',(12.7664342774515,1.67768005087614,1.1));
#13423=CARTESIAN_POINT('Ctrl Pts',(12.6856343728622,1.77018000694724,1.1));
#13424=CARTESIAN_POINT('Ctrl Pts',(12.70797027111,1.77258660535003,1.09999193474305));
#13425=CARTESIAN_POINT('Ctrl Pts',(12.7620607807224,1.75878051965913,1.09998076816122));
#13426=CARTESIAN_POINT('Ctrl Pts',(12.789311301819,1.70760782583852,1.09999039212455));
#13427=CARTESIAN_POINT('Ctrl Pts',(12.7895723566779,1.67768005087614,1.1));
#13428=CARTESIAN_POINT('Ctrl Pts',(12.6809355967604,1.81016478834023,1.08112516654061));
#13429=CARTESIAN_POINT('Ctrl Pts',(12.7128933108791,1.81335099699619,1.08149246505882));
#13430=CARTESIAN_POINT('Ctrl Pts',(12.7898658458254,1.7931743676233,1.08208124913004));
#13431=CARTESIAN_POINT('Ctrl Pts',(12.8289908274994,1.72043204305838,1.08173005449524));
#13432=CARTESIAN_POINT('Ctrl Pts',(12.829672543413,1.67768005087614,1.08128963884528));
#13433=CARTESIAN_POINT('Ctrl Pts',(12.6791127113589,1.82567684354491,1.04109086533338));
#13434=CARTESIAN_POINT('Ctrl Pts',(12.7147851087716,1.82957775596959,1.04203732134162));
#13435=CARTESIAN_POINT('Ctrl Pts',(12.8014031907485,1.80754024306994,1.04357783697133));
#13436=CARTESIAN_POINT('Ctrl Pts',(12.8450621014111,1.72550665092358,1.04265503156396));
#13437=CARTESIAN_POINT('Ctrl Pts',(12.8454164251054,1.67768005087614,1.0415166534692));
#13438=CARTESIAN_POINT('Ctrl Pts',(12.6790190612712,1.82647376985122,1.02368384096639));
#13439=CARTESIAN_POINT('Ctrl Pts',(12.7148414907177,1.83063166001164,1.02479882190871));
#13440=CARTESIAN_POINT('Ctrl Pts',(12.8023492944496,1.80880756543048,1.02662811038865));
#13441=CARTESIAN_POINT('Ctrl Pts',(12.8462542441509,1.7257797841646,1.02553011374107));
#13442=CARTESIAN_POINT('Ctrl Pts',(12.8463246402318,1.67768005087614,1.02418687649944));
#13443=CARTESIAN_POINT('',(12.7664342774515,1.67768005087614,1.1));
#13444=CARTESIAN_POINT('',(12.8463246402318,1.67768005087614,1.02418687649944));
#13445=CARTESIAN_POINT('Origin',(12.7664342774515,1.67768005087614,1.02));
#13446=CARTESIAN_POINT('',(12.6790190612712,1.82647376985123,1.02368384096637));
#13447=CARTESIAN_POINT('Ctrl Pts',(12.8463246402318,1.67768005087614,1.02418687649944));
#13448=CARTESIAN_POINT('Ctrl Pts',(12.8462542441509,1.7257797841646,1.02553011374107));
#13449=CARTESIAN_POINT('Ctrl Pts',(12.8023492944496,1.80880756543048,1.02662811038865));
#13450=CARTESIAN_POINT('Ctrl Pts',(12.7148414907177,1.83063166001164,1.02479882190871));
#13451=CARTESIAN_POINT('Ctrl Pts',(12.6790190612712,1.82647376985122,1.02368384096639));
#13452=CARTESIAN_POINT('',(12.6883460378814,1.74710477827991,1.1));
#13453=CARTESIAN_POINT('Origin',(12.6883460378814,1.74710477827991,1.02));
#13454=CARTESIAN_POINT('Ctrl Pts',(12.6883460378814,1.74710477827991,1.1));
#13455=CARTESIAN_POINT('Ctrl Pts',(12.7050904406715,1.74907248191433,1.1));
#13456=CARTESIAN_POINT('Ctrl Pts',(12.7459721545883,1.73893278412019,1.1));
#13457=CARTESIAN_POINT('Ctrl Pts',(12.7664342774515,1.70015954799943,1.1));
#13458=CARTESIAN_POINT('Ctrl Pts',(12.7664342774515,1.67768005087614,1.1));
#13459=CARTESIAN_POINT('Origin',(12.7664342774515,0.926416499322631,1.02));
#13460=CARTESIAN_POINT('',(12.7664342774515,-1.67768005087614,1.1));
#13461=CARTESIAN_POINT('',(12.8463246402318,-1.67768005087614,1.02418687649944));
#13462=CARTESIAN_POINT('Origin',(12.7664342774515,-1.67768005087614,1.02));
#13463=CARTESIAN_POINT('',(12.8463246402318,0.926416499322631,1.02418687649944));
#13464=CARTESIAN_POINT('',(12.7664342774515,0.926416499322631,1.1));
#13465=CARTESIAN_POINT('Ctrl Pts',(12.7664342774515,-1.67768005087614,1.1));
#13466=CARTESIAN_POINT('Ctrl Pts',(12.7664342774515,-1.69453967371875,1.1));
#13467=CARTESIAN_POINT('Ctrl Pts',(12.7515713182712,-1.73395715258217,1.1));
#13468=CARTESIAN_POINT('Ctrl Pts',(12.7106719082684,-1.74972838312583,1.1));
#13469=CARTESIAN_POINT('Ctrl Pts',(12.6883460378814,-1.74710477827991,1.1));
#13470=CARTESIAN_POINT('Ctrl Pts',(12.7895723566779,-1.67768005087614,1.1));
#13471=CARTESIAN_POINT('Ctrl Pts',(12.7893765655337,-1.70012588209812,1.09999279409341));
#13472=CARTESIAN_POINT('Ctrl Pts',(12.7694119126837,-1.75223468493452,1.09998162170574));
#13473=CARTESIAN_POINT('Ctrl Pts',(12.7154155705261,-1.77338880481765,1.09998924632407));
#13474=CARTESIAN_POINT('Ctrl Pts',(12.6856343728622,-1.77018000694724,1.1));
#13475=CARTESIAN_POINT('Ctrl Pts',(12.829672543413,-1.67768005087614,1.08128963884528));
#13476=CARTESIAN_POINT('Ctrl Pts',(12.8291612564778,-1.70974404501309,1.08161995058275));
#13477=CARTESIAN_POINT('Ctrl Pts',(12.800330508486,-1.78383870138124,1.08209231231141));
#13478=CARTESIAN_POINT('Ctrl Pts',(12.7235458822523,-1.81441306654821,1.08161489789823));
#13479=CARTESIAN_POINT('Ctrl Pts',(12.6809355967604,-1.81016478834023,1.08112516654061));
#13480=CARTESIAN_POINT('Ctrl Pts',(12.8454164251054,-1.67768005087614,1.0415166534692));
#13481=CARTESIAN_POINT('Ctrl Pts',(12.8451506823347,-1.71355000091203,1.04237043704028));
#13482=CARTESIAN_POINT('Ctrl Pts',(12.8132193893781,-1.79702133948082,1.04360777159741));
#13483=CARTESIAN_POINT('Ctrl Pts',(12.7266759079096,-1.8308780601112,1.04235280667771));
#13484=CARTESIAN_POINT('Ctrl Pts',(12.6791127113589,-1.82567684354491,1.04109086533338));
#13485=CARTESIAN_POINT('Ctrl Pts',(12.8463246402318,-1.67768005087614,1.02418687649944));
#13486=CARTESIAN_POINT('Ctrl Pts',(12.8462718431712,-1.71375485084279,1.02519430443067));
#13487=CARTESIAN_POINT('Ctrl Pts',(12.8143456047297,-1.79814359426379,1.02666431898144));
#13488=CARTESIAN_POINT('Ctrl Pts',(12.7267823005336,-1.83201762339849,1.02517048222283));
#13489=CARTESIAN_POINT('Ctrl Pts',(12.6790190612712,-1.82647376985122,1.02368384096639));
#13490=CARTESIAN_POINT('',(12.6883460378814,-1.74710477827991,1.1));
#13491=CARTESIAN_POINT('',(12.6790190612712,-1.82647376985122,1.02368384096639));
#13492=CARTESIAN_POINT('Origin',(12.6883460378814,-1.74710477827991,1.02));
#13493=CARTESIAN_POINT('Ctrl Pts',(12.6790190612712,-1.82647376985122,1.02368384096639));
#13494=CARTESIAN_POINT('Ctrl Pts',(12.7267823005336,-1.83201762339849,1.02517048222283));
#13495=CARTESIAN_POINT('Ctrl Pts',(12.8143456047297,-1.79814359426379,1.02666431898144));
#13496=CARTESIAN_POINT('Ctrl Pts',(12.8462718431712,-1.71375485084279,1.02519430443067));
#13497=CARTESIAN_POINT('Ctrl Pts',(12.8463246402318,-1.67768005087614,1.02418687649944));
#13498=CARTESIAN_POINT('Ctrl Pts',(12.7664342774515,-1.67768005087614,1.1));
#13499=CARTESIAN_POINT('Ctrl Pts',(12.7664342774515,-1.69453967371875,1.1));
#13500=CARTESIAN_POINT('Ctrl Pts',(12.7515713182712,-1.73395715258217,1.1));
#13501=CARTESIAN_POINT('Ctrl Pts',(12.7106719082684,-1.74972838312583,1.1));
#13502=CARTESIAN_POINT('Ctrl Pts',(12.6883460378814,-1.74710477827991,1.1));
#13503=CARTESIAN_POINT('Ctrl Pts',(12.6883460378814,-1.74710477827991,1.1));
#13504=CARTESIAN_POINT('Ctrl Pts',(10.9559705848985,-1.54352621428166,1.1));
#13505=CARTESIAN_POINT('Ctrl Pts',(6.89625808461774,-1.22619725057464,1.1));
#13506=CARTESIAN_POINT('Ctrl Pts',(2.82684345252479,-1.12583341467021,1.1));
#13507=CARTESIAN_POINT('Ctrl Pts',(0.501786340825443,-1.06996858265586,
1.1));
#13508=CARTESIAN_POINT('Ctrl Pts',(12.6856343728622,-1.77018000694724,1.1));
#13509=CARTESIAN_POINT('Ctrl Pts',(10.953864459251,-1.56662322149928,1.09999817462394));
#13510=CARTESIAN_POINT('Ctrl Pts',(6.89527069668598,-1.24931220526659,1.1000008953949));
#13511=CARTESIAN_POINT('Ctrl Pts',(2.8262782431937,-1.14895306774358,1.10000025453557));
#13512=CARTESIAN_POINT('Ctrl Pts',(0.501230998995504,-1.09308153985212,
1.1));
#13513=CARTESIAN_POINT('Ctrl Pts',(12.6809355941985,-1.8101648101409,1.08112518582372));
#13514=CARTESIAN_POINT('Ctrl Pts',(10.9502073547204,-1.60665097561358,1.08120831496985));
#13515=CARTESIAN_POINT('Ctrl Pts',(6.89356335983392,-1.28937229578717,1.08131090328882));
#13516=CARTESIAN_POINT('Ctrl Pts',(2.82529878789426,-1.18902174359502,1.08130951558098));
#13517=CARTESIAN_POINT('Ctrl Pts',(0.500268515819014,-1.13313944880305,
1.0813211979534));
#13518=CARTESIAN_POINT('Ctrl Pts',(12.6791127113589,-1.82567684354491,1.04109086533338));
#13519=CARTESIAN_POINT('Ctrl Pts',(10.9487809439014,-1.62227255850559,1.04130507278566));
#13520=CARTESIAN_POINT('Ctrl Pts',(6.89288912441654,-1.30512519378816,1.04157208078929));
#13521=CARTESIAN_POINT('Ctrl Pts',(2.82491362604336,-1.2047760518259,1.04156824165415));
#13522=CARTESIAN_POINT('Ctrl Pts',(0.499889770467655,-1.14890257814483,
1.04159845594383));
#13523=CARTESIAN_POINT('Ctrl Pts',(12.6790190612712,-1.82647376985122,1.02368384096639));
#13524=CARTESIAN_POINT('Ctrl Pts',(10.9487001718726,-1.62312516854374,1.02393618996614));
#13525=CARTESIAN_POINT('Ctrl Pts',(6.89285005483575,-1.30604661809728,1.02425267661394));
#13526=CARTESIAN_POINT('Ctrl Pts',(2.82489114035621,-1.20569670918473,1.0242479474763));
#13527=CARTESIAN_POINT('Ctrl Pts',(0.499867468581681,-1.14983076778971,
1.024283610038));
#13528=CARTESIAN_POINT('',(0.501786340825443,-1.06996858265586,1.1));
#13529=CARTESIAN_POINT('',(0.499867468607324,-1.1498307677904,1.02428361003669));
#13530=CARTESIAN_POINT('Origin',(0.501786340825443,-1.06996858265586,1.02));
#13531=CARTESIAN_POINT('Ctrl Pts',(0.499867468581681,-1.14983076778971,
1.024283610038));
#13532=CARTESIAN_POINT('Ctrl Pts',(2.82489114035621,-1.20569670918473,1.0242479474763));
#13533=CARTESIAN_POINT('Ctrl Pts',(6.89285005483575,-1.30604661809728,1.02425267661394));
#13534=CARTESIAN_POINT('Ctrl Pts',(10.9487001718726,-1.62312516854374,1.02393618996614));
#13535=CARTESIAN_POINT('Ctrl Pts',(12.6790190612712,-1.82647376985122,1.02368384096639));
#13536=CARTESIAN_POINT('Ctrl Pts',(12.6883460378814,-1.74710477827991,1.1));
#13537=CARTESIAN_POINT('Ctrl Pts',(10.9559705848985,-1.54352621428166,1.1));
#13538=CARTESIAN_POINT('Ctrl Pts',(6.89625808461774,-1.22619725057464,1.1));
#13539=CARTESIAN_POINT('Ctrl Pts',(2.82684345252479,-1.12583341467021,1.1));
#13540=CARTESIAN_POINT('Ctrl Pts',(0.501786340825443,-1.06996858265586,
1.1));
#13541=CARTESIAN_POINT('Ctrl Pts',(0.501786340845132,-1.06996858265633,
1.1));
#13542=CARTESIAN_POINT('Ctrl Pts',(0.486343670353271,-1.06959753705714,
1.1));
#13543=CARTESIAN_POINT('Ctrl Pts',(0.450546621606563,-1.05636265633066,
1.1));
#13544=CARTESIAN_POINT('Ctrl Pts',(0.4335657225485,-1.02068090721437,1.1));
#13545=CARTESIAN_POINT('Ctrl Pts',(0.433565722548536,-1.00008473726807,
1.1));
#13546=CARTESIAN_POINT('Ctrl Pts',(0.501230999004731,-1.09308153985199,
1.1));
#13547=CARTESIAN_POINT('Ctrl Pts',(0.480678852604012,-1.0924131923446,1.09999359215549));
#13548=CARTESIAN_POINT('Ctrl Pts',(0.433334506735602,-1.0746197149398,1.09998454864803));
#13549=CARTESIAN_POINT('Ctrl Pts',(0.410665947227687,-1.02750530853182,
1.09999122945172));
#13550=CARTESIAN_POINT('Ctrl Pts',(0.410427643322096,-1.00008473726803,
1.1));
#13551=CARTESIAN_POINT('Ctrl Pts',(0.500268097562941,-1.13315685597024,
1.08133662520967));
#13552=CARTESIAN_POINT('Ctrl Pts',(0.470917694462572,-1.13199579109467,
1.08163072487897));
#13553=CARTESIAN_POINT('Ctrl Pts',(0.403559863183325,-1.10627672518437,
1.08206304806334));
#13554=CARTESIAN_POINT('Ctrl Pts',(0.370932263602498,-1.0392553542177,1.08170715357768));
#13555=CARTESIAN_POINT('Ctrl Pts',(0.370309959289207,-1.00008473726796,
1.08130512018932));
#13556=CARTESIAN_POINT('Ctrl Pts',(0.4998897704516,-1.14890257814396,1.04159845594539));
#13557=CARTESIAN_POINT('Ctrl Pts',(0.467042111092653,-1.1478756708603,1.04235909019736));
#13558=CARTESIAN_POINT('Ctrl Pts',(0.391210771603448,-1.11942230347982,
1.04349095641912));
#13559=CARTESIAN_POINT('Ctrl Pts',(0.354907019248534,-1.04390490695311,
1.04255582181557));
#13560=CARTESIAN_POINT('Ctrl Pts',(0.354583574894623,-1.00008473726793,
1.04151665346919));
#13561=CARTESIAN_POINT('Ctrl Pts',(0.499867468565196,-1.14983076778922,
1.02428361003984));
#13562=CARTESIAN_POINT('Ctrl Pts',(0.466823083113769,-1.14898864521809,
1.02518140264794));
#13563=CARTESIAN_POINT('Ctrl Pts',(0.390185579422885,-1.12055776822857,
1.0265258196442));
#13564=CARTESIAN_POINT('Ctrl Pts',(0.353739620824501,-1.04415516223227,
1.0254130505005));
#13565=CARTESIAN_POINT('Ctrl Pts',(0.353675359768169,-1.00008473726793,
1.02418687649943));
#13566=CARTESIAN_POINT('',(0.433565722548536,-1.00008473726807,1.1));
#13567=CARTESIAN_POINT('',(0.353675359768456,-1.00008473726778,1.0241868765049));
#13568=CARTESIAN_POINT('Origin',(0.433565722548536,-1.00008473726807,1.02));
#13569=CARTESIAN_POINT('Ctrl Pts',(0.353675359768169,-1.00008473726793,
1.02418687649943));
#13570=CARTESIAN_POINT('Ctrl Pts',(0.353739620824501,-1.04415516223227,
1.0254130505005));
#13571=CARTESIAN_POINT('Ctrl Pts',(0.390185579422885,-1.12055776822857,
1.0265258196442));
#13572=CARTESIAN_POINT('Ctrl Pts',(0.466823083113769,-1.14898864521809,
1.02518140264794));
#13573=CARTESIAN_POINT('Ctrl Pts',(0.499867468565196,-1.14983076778922,
1.02428361003984));
#13574=CARTESIAN_POINT('Ctrl Pts',(0.501786340845132,-1.06996858265633,
1.1));
#13575=CARTESIAN_POINT('Ctrl Pts',(0.486343670353271,-1.06959753705714,
1.1));
#13576=CARTESIAN_POINT('Ctrl Pts',(0.450546621606563,-1.05636265633066,
1.1));
#13577=CARTESIAN_POINT('Ctrl Pts',(0.4335657225485,-1.02068090721437,1.1));
#13578=CARTESIAN_POINT('Ctrl Pts',(0.433565722548536,-1.00008473726807,
1.1));
#13579=CARTESIAN_POINT('Origin',(0.433565722548535,-0.576416499322632,1.02));
#13580=CARTESIAN_POINT('',(0.433565722548535,1.0000847372682,1.1));
#13581=CARTESIAN_POINT('',(0.35367535976817,1.0000847372682,1.02418687649944));
#13582=CARTESIAN_POINT('Origin',(0.433565722548535,1.0000847372682,1.02));
#13583=CARTESIAN_POINT('',(0.35367535976817,-0.576416499322632,1.02418687649944));
#13584=CARTESIAN_POINT('',(0.433565722548535,-0.576416499322632,1.1));
#13585=CARTESIAN_POINT('Ctrl Pts',(0.433565722548535,1.0000847372682,1.1));
#13586=CARTESIAN_POINT('Ctrl Pts',(0.433565722548535,1.01553186472631,1.1));
#13587=CARTESIAN_POINT('Ctrl Pts',(0.445933851022605,1.05163704585376,1.1));
#13588=CARTESIAN_POINT('Ctrl Pts',(0.481196113556474,1.06947385520094,1.1));
#13589=CARTESIAN_POINT('Ctrl Pts',(0.501786340877041,1.0699685826571,1.1));
#13590=CARTESIAN_POINT('Ctrl Pts',(0.410427643322096,1.0000847372682,1.1));
#13591=CARTESIAN_POINT('Ctrl Pts',(0.410606371251307,1.0206501657139,1.09999342208879));
#13592=CARTESIAN_POINT('Ctrl Pts',(0.427269489276852,1.06840883688971,1.09998438534344));
#13593=CARTESIAN_POINT('Ctrl Pts',(0.473828137181897,1.09219040985597,1.09999145620732));
#13594=CARTESIAN_POINT('Ctrl Pts',(0.501230999047159,1.09308153985336,1.1));
#13595=CARTESIAN_POINT('Ctrl Pts',(0.370309959289211,1.0000847372682,1.08130512018932));
#13596=CARTESIAN_POINT('Ctrl Pts',(0.370776687524182,1.02946269997745,1.08160664523056));
#13597=CARTESIAN_POINT('Ctrl Pts',(0.394906927696186,1.09741901043509,1.08206104999852));
#13598=CARTESIAN_POINT('Ctrl Pts',(0.461134226826275,1.13160876948958,1.08172875810162));
#13599=CARTESIAN_POINT('Ctrl Pts',(0.500268097623607,1.13315685597264,1.08133662520906));
#13600=CARTESIAN_POINT('Ctrl Pts',(0.354583574894625,1.0000847372682,1.0415166534692));
#13601=CARTESIAN_POINT('Ctrl Pts',(0.354826158160091,1.03294986452867,1.0422960297289));
#13602=CARTESIAN_POINT('Ctrl Pts',(0.381463759848658,1.10944036955345,1.04348552759116));
#13603=CARTESIAN_POINT('Ctrl Pts',(0.456092891378057,1.14753336845448,1.04261263494683));
#13604=CARTESIAN_POINT('Ctrl Pts',(0.499889770519448,1.14890257814608,1.04159845594382));
#13605=CARTESIAN_POINT('Ctrl Pts',(0.35367535976817,1.0000847372682,1.02418687649944));
#13606=CARTESIAN_POINT('Ctrl Pts',(0.353723555560473,1.03313755598801,1.02510650700014));
#13607=CARTESIAN_POINT('Ctrl Pts',(0.380300727059747,1.11043180383933,1.02651925632578));
#13608=CARTESIAN_POINT('Ctrl Pts',(0.455808288035698,1.1487079377163,1.02548066684923));
#13609=CARTESIAN_POINT('Ctrl Pts',(0.499867468633476,1.14983076779096,1.02428361003799));
#13610=CARTESIAN_POINT('',(0.501786340877041,1.0699685826571,1.1));
#13611=CARTESIAN_POINT('',(0.499867468633699,1.14983076779054,1.0242836100458));
#13612=CARTESIAN_POINT('Origin',(0.501786340877041,1.0699685826571,1.02));
#13613=CARTESIAN_POINT('Ctrl Pts',(0.499867468633476,1.14983076779096,1.02428361003799));
#13614=CARTESIAN_POINT('Ctrl Pts',(0.455808288035698,1.1487079377163,1.02548066684923));
#13615=CARTESIAN_POINT('Ctrl Pts',(0.380300727059747,1.11043180383933,1.02651925632578));
#13616=CARTESIAN_POINT('Ctrl Pts',(0.353723555560473,1.03313755598801,1.02510650700014));
#13617=CARTESIAN_POINT('Ctrl Pts',(0.35367535976817,1.0000847372682,1.02418687649944));
#13618=CARTESIAN_POINT('Ctrl Pts',(0.433565722548535,1.0000847372682,1.1));
#13619=CARTESIAN_POINT('Ctrl Pts',(0.433565722548535,1.01553186472631,1.1));
#13620=CARTESIAN_POINT('Ctrl Pts',(0.445933851022605,1.05163704585376,1.1));
#13621=CARTESIAN_POINT('Ctrl Pts',(0.481196113556474,1.06947385520094,1.1));
#13622=CARTESIAN_POINT('Ctrl Pts',(0.501786340877041,1.0699685826571,1.1));
#13623=CARTESIAN_POINT('Ctrl Pts',(0.501786340877248,1.0699685826571,1.1));
#13624=CARTESIAN_POINT('Ctrl Pts',(2.82684356715236,1.12583341742443,1.1));
#13625=CARTESIAN_POINT('Ctrl Pts',(6.89625445951469,1.22619710828032,1.1));
#13626=CARTESIAN_POINT('Ctrl Pts',(10.9559704995293,1.54352620424957,1.1));
#13627=CARTESIAN_POINT('Ctrl Pts',(12.6883460378814,1.74710477827991,1.1));
#13628=CARTESIAN_POINT('Ctrl Pts',(0.501230999047308,1.09308153985337,1.1));
#13629=CARTESIAN_POINT('Ctrl Pts',(2.82627835782077,1.14895307049812,1.10000025453558));
#13630=CARTESIAN_POINT('Ctrl Pts',(6.89526707210341,1.24931206297629,1.10000089539479));
#13631=CARTESIAN_POINT('Ctrl Pts',(10.9538643739116,1.56662321146826,1.09999817462385));
#13632=CARTESIAN_POINT('Ctrl Pts',(12.6856343728622,1.77018000694724,1.1));
#13633=CARTESIAN_POINT('Ctrl Pts',(0.500268515870817,1.1331394488043,1.0813211979534));
#13634=CARTESIAN_POINT('Ctrl Pts',(2.82529890252049,1.18902174635009,1.08130951558041));
#13635=CARTESIAN_POINT('Ctrl Pts',(6.89355973615254,1.28937215350496,1.08131090331441));
#13636=CARTESIAN_POINT('Ctrl Pts',(10.9502072694324,1.60665096558469,1.08120831497395));
#13637=CARTESIAN_POINT('Ctrl Pts',(12.6809355941985,1.8101648101409,1.08112518582372));
#13638=CARTESIAN_POINT('Ctrl Pts',(0.499889770519458,1.14890257814608,1.04159845594383));
#13639=CARTESIAN_POINT('Ctrl Pts',(2.82491374066927,1.20477605458053,1.04156824165266));
#13640=CARTESIAN_POINT('Ctrl Pts',(6.89288550108907,1.30512505153819,1.04157208085565));
#13641=CARTESIAN_POINT('Ctrl Pts',(10.948780858633,1.62227254848209,1.04130507279621));
#13642=CARTESIAN_POINT('Ctrl Pts',(12.6791127113589,1.82567684354491,1.04109086533338));
#13643=CARTESIAN_POINT('Ctrl Pts',(0.499867468633484,1.14983076779096,1.024283610038));
#13644=CARTESIAN_POINT('Ctrl Pts',(2.82489125498211,1.205696711939,1.02424794747454));
#13645=CARTESIAN_POINT('Ctrl Pts',(6.89284643152835,1.3060464758645,1.02425267669241));
#13646=CARTESIAN_POINT('Ctrl Pts',(10.9487000866048,1.62312515852299,1.02393618997858));
#13647=CARTESIAN_POINT('Ctrl Pts',(12.6790190612712,1.82647376985123,1.02368384096639));
#13648=CARTESIAN_POINT('Ctrl Pts',(12.6790190612712,1.82647376985123,1.02368384096639));
#13649=CARTESIAN_POINT('Ctrl Pts',(10.9487000866048,1.62312515852299,1.02393618997858));
#13650=CARTESIAN_POINT('Ctrl Pts',(6.89284643152835,1.3060464758645,1.02425267669241));
#13651=CARTESIAN_POINT('Ctrl Pts',(2.82489125498211,1.205696711939,1.02424794747454));
#13652=CARTESIAN_POINT('Ctrl Pts',(0.499867468633484,1.14983076779096,1.024283610038));
#13653=CARTESIAN_POINT('Ctrl Pts',(0.501786340877248,1.0699685826571,1.1));
#13654=CARTESIAN_POINT('Ctrl Pts',(2.82684356715236,1.12583341742443,1.1));
#13655=CARTESIAN_POINT('Ctrl Pts',(6.89625445951469,1.22619710828032,1.1));
#13656=CARTESIAN_POINT('Ctrl Pts',(10.9559704995293,1.54352620424957,1.1));
#13657=CARTESIAN_POINT('Ctrl Pts',(12.6883460378814,1.74710477827991,1.1));
#13658=CARTESIAN_POINT('Origin',(0.347167001354737,-1.15283299864526,0.9));
#13659=CARTESIAN_POINT('',(0.347167001354737,1.00658943961019,0.9));
#13660=CARTESIAN_POINT('Ctrl Pts',(0.347167001354737,1.00658943961019,0.9));
#13661=CARTESIAN_POINT('Ctrl Pts',(0.349336454155793,1.00442120424608,0.941395625434512));
#13662=CARTESIAN_POINT('Ctrl Pts',(0.351505906960267,1.0022529701308,0.982791250934257));
#13663=CARTESIAN_POINT('Ctrl Pts',(0.35367535976817,1.0000847372682,1.02418687649944));
#13664=CARTESIAN_POINT('',(0.347167001354737,-1.00658943961019,0.9));
#13665=CARTESIAN_POINT('',(0.347167001354737,-1.15283299864526,0.9));
#13666=CARTESIAN_POINT('Ctrl Pts',(0.353675359768457,-1.00008473726791,
1.02418687650491));
#13667=CARTESIAN_POINT('Ctrl Pts',(0.351505906960458,-1.0022529701306,0.982791250937906));
#13668=CARTESIAN_POINT('Ctrl Pts',(0.349336454155888,-1.00442120424599,
0.941395625436337));
#13669=CARTESIAN_POINT('Ctrl Pts',(0.347167001354737,-1.00658943961019,
0.900000000000001));
#13670=CARTESIAN_POINT('Ctrl Pts',(0.346996296805428,1.00676004836741,0.896742763161407));
#13671=CARTESIAN_POINT('Ctrl Pts',(0.349222651122738,1.0045349433512,0.939224134205317));
#13672=CARTESIAN_POINT('Ctrl Pts',(0.351449005443648,1.00230983965007,0.981705505317921));
#13673=CARTESIAN_POINT('Ctrl Pts',(0.35367535976817,1.0000847372682,1.02418687649944));
#13674=CARTESIAN_POINT('Ctrl Pts',(0.347116900426942,1.05081591929015,0.899044017348554));
#13675=CARTESIAN_POINT('Ctrl Pts',(0.349343263597644,1.04859056550012,0.941525373982715));
#13676=CARTESIAN_POINT('Ctrl Pts',(0.351569598045448,1.04636522758029,0.98400673296308));
#13677=CARTESIAN_POINT('Ctrl Pts',(0.353795961241832,1.04413987589222,1.02648808970312));
#13678=CARTESIAN_POINT('Ctrl Pts',(0.383592239441417,1.12715274970112,0.901130824661994));
#13679=CARTESIAN_POINT('Ctrl Pts',(0.38581816402279,1.12492699736917,0.943612181832344));
#13680=CARTESIAN_POINT('Ctrl Pts',(0.388044096297176,1.12270123909217,0.986093538279035));
#13681=CARTESIAN_POINT('Ctrl Pts',(0.390270019973987,1.12047548800691,1.02857489555427));
#13682=CARTESIAN_POINT('Ctrl Pts',(0.460164343209507,1.15561854687756,0.898608842835867));
#13683=CARTESIAN_POINT('Ctrl Pts',(0.462389604568499,1.15339312775892,0.941090251624243));
#13684=CARTESIAN_POINT('Ctrl Pts',(0.464614871986574,1.15116771740584,0.983571660556392));
#13685=CARTESIAN_POINT('Ctrl Pts',(0.466840131020026,1.14894230022584,1.02605306955844));
#13686=CARTESIAN_POINT('Ctrl Pts',(0.493196683694039,1.15650174777388,0.896923951850831));
#13687=CARTESIAN_POINT('Ctrl Pts',(0.49542175781822,1.15427660869429,0.939405385103827));
#13688=CARTESIAN_POINT('Ctrl Pts',(0.497646830577711,1.15205147087705,0.981886818489558));
#13689=CARTESIAN_POINT('Ctrl Pts',(0.499871901968125,1.1498263343261,1.02436825200844));
#13690=CARTESIAN_POINT('',(0.493357799610229,1.15634062715414,0.9));
#13691=CARTESIAN_POINT('Ctrl Pts',(0.499867468633513,1.14983076779054,1.02428361004581));
#13692=CARTESIAN_POINT('Ctrl Pts',(0.497697580259738,1.1520007197087,0.982855739904038));
#13693=CARTESIAN_POINT('Ctrl Pts',(0.495527690583954,1.15417067283112,0.941427869888898));
#13694=CARTESIAN_POINT('Ctrl Pts',(0.493357799610229,1.15634062715414,0.9));
#13695=CARTESIAN_POINT('Ctrl Pts',(0.493357799610229,1.15634062715414,0.9));
#13696=CARTESIAN_POINT('Ctrl Pts',(0.482602647031033,1.1560824793541,0.899999999999731));
#13697=CARTESIAN_POINT('Ctrl Pts',(0.471926867235344,1.1546337250523,0.899998382330426));
#13698=CARTESIAN_POINT('Ctrl Pts',(0.461511103461674,1.15208577142905,0.899997935562642));
#13699=CARTESIAN_POINT('Ctrl Pts',(0.453002267216956,1.15000429947842,0.899997570589511));
#13700=CARTESIAN_POINT('Ctrl Pts',(0.444666263429443,1.14718801542572,0.899997957558805));
#13701=CARTESIAN_POINT('Ctrl Pts',(0.436607964282466,1.14366186386534,0.899998978246166));
#13702=CARTESIAN_POINT('Ctrl Pts',(0.426757323168539,1.13935141908028,0.900000225956719));
#13703=CARTESIAN_POINT('Ctrl Pts',(0.417425277328103,1.13402704260718,0.900002535631972));
#13704=CARTESIAN_POINT('Ctrl Pts',(0.408793513884033,1.1277570068973,0.900002417864976));
#13705=CARTESIAN_POINT('Ctrl Pts',(0.406442206080559,1.1260490379535,0.900002385785035));
#13706=CARTESIAN_POINT('Ctrl Pts',(0.404142986411405,1.12427063023042,0.900002152965402));
#13707=CARTESIAN_POINT('Ctrl Pts',(0.40189988757483,1.12242258952304,0.900001599918915));
#13708=CARTESIAN_POINT('Ctrl Pts',(0.397433290854798,1.11874265691041,0.900000498658648));
#13709=CARTESIAN_POINT('Ctrl Pts',(0.393188994678067,1.11478677136369,0.899998147353889));
#13710=CARTESIAN_POINT('Ctrl Pts',(0.389180227688998,1.11057998277971,0.899995556820878));
#13711=CARTESIAN_POINT('Ctrl Pts',(0.381747711834384,1.10278032195316,0.899990753803459));
#13712=CARTESIAN_POINT('Ctrl Pts',(0.375201641992584,1.09420365251288,0.899985427555825));
#13713=CARTESIAN_POINT('Ctrl Pts',(0.369602030462105,1.08503231460429,0.899982994308828));
#13714=CARTESIAN_POINT('Ctrl Pts',(0.365103987453251,1.07766518348509,0.899981039735804));
#13715=CARTESIAN_POINT('Ctrl Pts',(0.361217082581294,1.06991300661492,0.899980859474918));
#13716=CARTESIAN_POINT('Ctrl Pts',(0.357992910300892,1.06185737523451,0.899982473761482));
#13717=CARTESIAN_POINT('Ctrl Pts',(0.354005020049728,1.0518935857546,0.899984470428251));
#13718=CARTESIAN_POINT('Ctrl Pts',(0.351071168910505,1.04156966067519,0.899989252895565));
#13719=CARTESIAN_POINT('Ctrl Pts',(0.349267161175031,1.03104850244781,0.899993624760896));
#13720=CARTESIAN_POINT('Ctrl Pts',(0.347885225415831,1.022988911296,0.899996973769283));
#13721=CARTESIAN_POINT('Ctrl Pts',(0.347167001481006,1.014812725533,0.899999999989923));
#13722=CARTESIAN_POINT('Ctrl Pts',(0.347167001354737,1.00658943961019,0.900000000000001));
#13723=CARTESIAN_POINT('Ctrl Pts',(0.493357799610229,1.15634062715414,0.9));
#13724=CARTESIAN_POINT('Ctrl Pts',(0.495478181125715,1.15416948447463,0.941427870236244));
#13725=CARTESIAN_POINT('Ctrl Pts',(0.4975985626412,1.15199834179512,0.982855740472488));
#13726=CARTESIAN_POINT('Ctrl Pts',(0.499718944156686,1.14982719911562,1.02428361070873));
#13727=CARTESIAN_POINT('Ctrl Pts',(4.55741138981048,1.2538870134557,0.9));
#13728=CARTESIAN_POINT('Ctrl Pts',(4.55812062853622,1.25171587077619,0.941427870236244));
#13729=CARTESIAN_POINT('Ctrl Pts',(4.55882986726197,1.24954472809669,0.982855740472489));
#13730=CARTESIAN_POINT('Ctrl Pts',(4.55953910598771,1.24737358541718,1.02428361070873));
#13731=CARTESIAN_POINT('Ctrl Pts',(8.62146498001072,1.3558778793304,0.9));
#13732=CARTESIAN_POINT('Ctrl Pts',(8.62076307594673,1.35370673665089,0.941427870236244));
#13733=CARTESIAN_POINT('Ctrl Pts',(8.62006117188274,1.35153559397139,0.982855740472488));
#13734=CARTESIAN_POINT('Ctrl Pts',(8.61935926781874,1.34936445129188,1.02428361070873));
#13735=CARTESIAN_POINT('Ctrl Pts',(12.685518570211,1.83297820604925,0.9));
#13736=CARTESIAN_POINT('Ctrl Pts',(12.6834055233572,1.83080706336974,0.941427870236244));
#13737=CARTESIAN_POINT('Ctrl Pts',(12.6812924765035,1.82863592069023,0.982855740472488));
#13738=CARTESIAN_POINT('Ctrl Pts',(12.6791794296498,1.82646477801072,1.02428361070873));
#13739=CARTESIAN_POINT('',(12.685518570211,1.83297820604925,0.9));
#13740=CARTESIAN_POINT('Ctrl Pts',(12.685518570211,1.83297820604925,0.9));
#13741=CARTESIAN_POINT('Ctrl Pts',(12.6833520729681,1.83081006895277,0.941227947697879));
#13742=CARTESIAN_POINT('Ctrl Pts',(12.6811855699938,1.8286419235626,0.982455894687412));
#13743=CARTESIAN_POINT('Ctrl Pts',(12.6790190612712,1.82647376985122,1.02368384096639));
#13744=CARTESIAN_POINT('Ctrl Pts',(0.493357799610229,1.15634062715414,0.9));
#13745=CARTESIAN_POINT('Ctrl Pts',(4.55741138981048,1.2538870134557,0.9));
#13746=CARTESIAN_POINT('Ctrl Pts',(8.62146498001073,1.3558778793304,0.9));
#13747=CARTESIAN_POINT('Ctrl Pts',(12.685518570211,1.83297820604925,0.9));
#13748=CARTESIAN_POINT('Ctrl Pts',(12.6857396223418,1.83319942548878,0.895793428058847));
#13749=CARTESIAN_POINT('Ctrl Pts',(12.6834994414517,1.83095754915284,0.938423566452776));
#13750=CARTESIAN_POINT('Ctrl Pts',(12.6812592544344,1.82871566395046,0.981053704089438));
#13751=CARTESIAN_POINT('Ctrl Pts',(12.6790190612712,1.82647376985122,1.02368384096639));
#13752=CARTESIAN_POINT('Ctrl Pts',(12.7096132738247,1.83593722009608,0.897188525535458));
#13753=CARTESIAN_POINT('Ctrl Pts',(12.7073735515623,1.83369637734113,0.939818742641338));
#13754=CARTESIAN_POINT('Ctrl Pts',(12.7051338254027,1.83145551796363,0.982448958687984));
#13755=CARTESIAN_POINT('Ctrl Pts',(12.7028940916787,1.82921465970329,1.02507917444001));
#13756=CARTESIAN_POINT('Ctrl Pts',(12.7586310095219,1.82964538228831,0.8994266592275));
#13757=CARTESIAN_POINT('Ctrl Pts',(12.7563927428119,1.82740607701793,0.942057032676437));
#13758=CARTESIAN_POINT('Ctrl Pts',(12.7541544559015,1.82516675428928,0.984687404166494));
#13759=CARTESIAN_POINT('Ctrl Pts',(12.7519161806021,1.82292743696394,1.02731777659207));
#13760=CARTESIAN_POINT('Ctrl Pts',(12.8300025526753,1.78023902864912,0.90056967297836));
#13761=CARTESIAN_POINT('Ctrl Pts',(12.8277672375473,1.7780001144899,0.943200215636435));
#13762=CARTESIAN_POINT('Ctrl Pts',(12.8255319263559,1.7757611919149,0.985830758073823));
#13763=CARTESIAN_POINT('Ctrl Pts',(12.8232966088089,1.77352226682369,1.02846130007111));
#13764=CARTESIAN_POINT('Ctrl Pts',(12.8529050075203,1.72043671272769,0.898625988813541));
#13765=CARTESIAN_POINT('Ctrl Pts',(12.8506708576607,1.71819639833573,0.941256511626846));
#13766=CARTESIAN_POINT('Ctrl Pts',(12.8484366444933,1.71595605563573,0.983887029620282));
#13767=CARTESIAN_POINT('Ctrl Pts',(12.8462024947189,1.71371572743615,1.0265175517275));
#13768=CARTESIAN_POINT('Ctrl Pts',(12.853004077605,1.68438049200639,0.896735618985435));
#13769=CARTESIAN_POINT('Ctrl Pts',(12.8507699092581,1.68213930602179,0.939366090596142));
#13770=CARTESIAN_POINT('Ctrl Pts',(12.8485357409326,1.67989811224666,0.981996561798403));
#13771=CARTESIAN_POINT('Ctrl Pts',(12.8463015726285,1.67765691065502,1.02462703259085));
#13772=CARTESIAN_POINT('',(12.8528329986453,1.6842088756636,0.9));
#13773=CARTESIAN_POINT('Ctrl Pts',(12.8463246402318,1.67768005087614,1.02418687649944));
#13774=CARTESIAN_POINT('Ctrl Pts',(12.8484940930161,1.67985633316752,0.982791251385616));
#13775=CARTESIAN_POINT('Ctrl Pts',(12.8506635458206,1.68203260808875,0.941395625885387));
#13776=CARTESIAN_POINT('Ctrl Pts',(12.8528329986453,1.6842088756636,0.9));
#13777=CARTESIAN_POINT('Ctrl Pts',(12.8528329986453,1.6842088756636,0.900000000000001));
#13778=CARTESIAN_POINT('Ctrl Pts',(12.8528329990894,1.69496116035511,0.900000000031321));
#13779=CARTESIAN_POINT('Ctrl Pts',(12.8516279916809,1.7056415234076,0.899996564780585));
#13780=CARTESIAN_POINT('Ctrl Pts',(12.8493173682463,1.71608623918215,0.899994054968391));
#13781=CARTESIAN_POINT('Ctrl Pts',(12.847426586744,1.72463314262321,0.89999200119087));
#13782=CARTESIAN_POINT('Ctrl Pts',(12.8447941883809,1.73302290492875,0.899990534206534));
#13783=CARTESIAN_POINT('Ctrl Pts',(12.8414494901174,1.74115996769839,0.899990418365756));
#13784=CARTESIAN_POINT('Ctrl Pts',(12.8373567881217,1.75111679202539,0.899990276618506));
#13785=CARTESIAN_POINT('Ctrl Pts',(12.8322422209112,1.76059035368083,0.899992293328656));
#13786=CARTESIAN_POINT('Ctrl Pts',(12.8261823199623,1.76941466903515,0.899994578235276));
#13787=CARTESIAN_POINT('Ctrl Pts',(12.8228443945912,1.77427529404419,0.899995836811587));
#13788=CARTESIAN_POINT('Ctrl Pts',(12.819218773978,1.77893868154471,0.899997117508201));
#13789=CARTESIAN_POINT('Ctrl Pts',(12.8153125401773,1.78337342370743,0.899997612422461));
#13790=CARTESIAN_POINT('Ctrl Pts',(12.8134661485928,1.78546962967624,0.899997846357645));
#13791=CARTESIAN_POINT('Ctrl Pts',(12.8115570049875,1.7875146981109,0.899997899028016));
#13792=CARTESIAN_POINT('Ctrl Pts',(12.8095877759185,1.78950657520057,0.899997852068527));
#13793=CARTESIAN_POINT('Ctrl Pts',(12.802037518393,1.7971436679198,0.899997672020282));
#13794=CARTESIAN_POINT('Ctrl Pts',(12.7936869960543,1.80392089040634,0.899996345477631));
#13795=CARTESIAN_POINT('Ctrl Pts',(12.7847141304683,1.80975200096328,0.89999606036814));
#13796=CARTESIAN_POINT('Ctrl Pts',(12.7774211187199,1.81449144093269,0.899995828635385));
#13797=CARTESIAN_POINT('Ctrl Pts',(12.7697156358622,1.81860556854039,0.899996199361957));
#13798=CARTESIAN_POINT('Ctrl Pts',(12.761679297021,1.82202698480181,0.89999650903244));
#13799=CARTESIAN_POINT('Ctrl Pts',(12.7599722005109,1.82275376945776,0.899996574813315));
#13800=CARTESIAN_POINT('Ctrl Pts',(12.7582527406357,1.82344811243542,0.899996631272027));
#13801=CARTESIAN_POINT('Ctrl Pts',(12.7565217796305,1.82410952822173,0.899996662852262));
#13802=CARTESIAN_POINT('Ctrl Pts',(12.7461353325744,1.82807828316523,0.899996852346099));
#13803=CARTESIAN_POINT('Ctrl Pts',(12.7353361797362,1.83086624339127,0.899996468077086));
#13804=CARTESIAN_POINT('Ctrl Pts',(12.7243231747362,1.83245001845531,0.899997092905297));
#13805=CARTESIAN_POINT('Ctrl Pts',(12.713718016754,1.83397514123175,0.899997694594108));
#13806=CARTESIAN_POINT('Ctrl Pts',(12.702988146695,1.83437268605832,0.899999174299692));
#13807=CARTESIAN_POINT('Ctrl Pts',(12.6923097158784,1.83361665751845,0.899999788491474));
#13808=CARTESIAN_POINT('Ctrl Pts',(12.6900431251392,1.83345618381998,0.899999918859074));
#13809=CARTESIAN_POINT('Ctrl Pts',(12.6877788433122,1.83324355125563,0.900000000001074));
#13810=CARTESIAN_POINT('Ctrl Pts',(12.685518570211,1.83297820604925,0.9));
#13811=CARTESIAN_POINT('Origin',(6.88201982834292,-2.22044604925031E-16,
1.1));
#13812=CARTESIAN_POINT('Origin',(12.8528329986453,1.85283299864526,0.9));
#13813=CARTESIAN_POINT('',(12.8528329986453,-1.6842088756636,0.9));
#13814=CARTESIAN_POINT('Ctrl Pts',(12.8528329986453,-1.6842088756636,0.9));
#13815=CARTESIAN_POINT('Ctrl Pts',(12.8506635458206,-1.68203260808875,0.941395625885387));
#13816=CARTESIAN_POINT('Ctrl Pts',(12.8484940930161,-1.67985633316752,0.982791251385615));
#13817=CARTESIAN_POINT('Ctrl Pts',(12.8463246402318,-1.67768005087614,1.02418687649944));
#13818=CARTESIAN_POINT('',(12.8528329986453,1.85283299864526,0.9));
#13819=CARTESIAN_POINT('Ctrl Pts',(0.49319751180194,-1.1565009196418,0.896939762205254));
#13820=CARTESIAN_POINT('Ctrl Pts',(0.495422309889911,-1.15427605660646,
0.939415925341967));
#13821=CARTESIAN_POINT('Ctrl Pts',(0.49764710661353,-1.15205119483315,0.981892088611382));
#13822=CARTESIAN_POINT('Ctrl Pts',(0.499871901968411,-1.14982633432581,
1.02436825201392));
#13823=CARTESIAN_POINT('Ctrl Pts',(0.449154391250001,-1.15532331830903,
0.899186283506502));
#13824=CARTESIAN_POINT('Ctrl Pts',(0.451379443529967,-1.1530980743259,0.94166241338335));
#13825=CARTESIAN_POINT('Ctrl Pts',(0.453604490603533,-1.15087286444957,
0.984138545342204));
#13826=CARTESIAN_POINT('Ctrl Pts',(0.45582954070428,-1.14864762219213,1.02661467541392));
#13827=CARTESIAN_POINT('Ctrl Pts',(0.373709798968055,-1.1170292567097,0.901134386478875));
#13828=CARTESIAN_POINT('Ctrl Pts',(0.37593556973194,-1.11480381901192,0.943610469359475));
#13829=CARTESIAN_POINT('Ctrl Pts',(0.378161343437362,-1.11257837175868,
0.98608655157339));
#13830=CARTESIAN_POINT('Ctrl Pts',(0.380387113556173,-1.11035293539114,
1.02856263455032));
#13831=CARTESIAN_POINT('Ctrl Pts',(0.347087578105715,-1.039801123372,0.898484514129229));
#13832=CARTESIAN_POINT('Ctrl Pts',(0.349313658773859,-1.03757611304936,
0.940960604750146));
#13833=CARTESIAN_POINT('Ctrl Pts',(0.351539730193144,-1.03535109931323,
0.983436695671939));
#13834=CARTESIAN_POINT('Ctrl Pts',(0.353765810873703,-1.03312609123593,
1.02591278640767));
#13835=CARTESIAN_POINT('Ctrl Pts',(0.346997125389779,-1.00675922024802,
0.896758573492677));
#13836=CARTESIAN_POINT('Ctrl Pts',(0.349223203512402,-1.00453439127183,
0.939234674428006));
#13837=CARTESIAN_POINT('Ctrl Pts',(0.351449281638624,-1.0023095636104,0.98171077543201));
#13838=CARTESIAN_POINT('Ctrl Pts',(0.353675359768457,-1.00008473726791,
1.02418687650491));
#13839=CARTESIAN_POINT('',(0.493357799610228,-1.15634062715414,0.9));
#13840=CARTESIAN_POINT('Ctrl Pts',(0.347167001354737,-1.00658943961019,
0.900000000000001));
#13841=CARTESIAN_POINT('Ctrl Pts',(0.347167001425373,-1.01734828759763,
0.899999999998142));
#13842=CARTESIAN_POINT('Ctrl Pts',(0.348359077578701,-1.02805639415283,
0.899998433630397));
#13843=CARTESIAN_POINT('Ctrl Pts',(0.350656214310366,-1.0385309656087,0.899998024549738));
#13844=CARTESIAN_POINT('Ctrl Pts',(0.352533324612331,-1.04709028457193,
0.899997690268584));
#13845=CARTESIAN_POINT('Ctrl Pts',(0.355149562279486,-1.05549438497634,
0.899998101733499));
#13846=CARTESIAN_POINT('Ctrl Pts',(0.358482507184576,-1.0636377229308,0.899999127793999));
#13847=CARTESIAN_POINT('Ctrl Pts',(0.362555301547827,-1.07358872478153,
0.900000381620131));
#13848=CARTESIAN_POINT('Ctrl Pts',(0.367654000430903,-1.08304569392442,
0.900002668831236));
#13849=CARTESIAN_POINT('Ctrl Pts',(0.373714802804109,-1.09182534802447,
0.900002509451715));
#13850=CARTESIAN_POINT('Ctrl Pts',(0.375364773372187,-1.09421548879643,
0.90000246606282));
#13851=CARTESIAN_POINT('Ctrl Pts',(0.377086318771695,-1.09655531312597,
0.900002220932131));
#13852=CARTESIAN_POINT('Ctrl Pts',(0.378878733123435,-1.0988407769929,0.900001655250762));
#13853=CARTESIAN_POINT('Ctrl Pts',(0.382452759797804,-1.10339793132263,
0.900000527297116));
#13854=CARTESIAN_POINT('Ctrl Pts',(0.386308400219556,-1.10773917492176,
0.899998144709029));
#13855=CARTESIAN_POINT('Ctrl Pts',(0.390420886280218,-1.11185064093822,
0.899995523300098));
#13856=CARTESIAN_POINT('Ctrl Pts',(0.398040323803163,-1.11946818856709,
0.899990666466232));
#13857=CARTESIAN_POINT('Ctrl Pts',(0.406457812610252,-1.12621813960646,
0.899985292057237));
#13858=CARTESIAN_POINT('Ctrl Pts',(0.41549254786509,-1.13203603704298,0.899982834497606));
#13859=CARTESIAN_POINT('Ctrl Pts',(0.422749169000726,-1.13670892189372,
0.899980860606988));
#13860=CARTESIAN_POINT('Ctrl Pts',(0.430405328105449,-1.14078012415116,
0.899980677151631));
#13861=CARTESIAN_POINT('Ctrl Pts',(0.438380728308649,-1.14419607025517,
0.899982305341352));
#13862=CARTESIAN_POINT('Ctrl Pts',(0.448245442291908,-1.14842122892304,
0.899984319237269));
#13863=CARTESIAN_POINT('Ctrl Pts',(0.458495412124849,-1.1516012547891,0.899989147510445));
#13864=CARTESIAN_POINT('Ctrl Pts',(0.468969635281765,-1.1536564168707,0.899993562691215));
#13865=CARTESIAN_POINT('Ctrl Pts',(0.476989372009021,-1.15522998071208,
0.899996943236659));
#13866=CARTESIAN_POINT('Ctrl Pts',(0.485141446557615,-1.15614341614473,
0.89999999999177));
#13867=CARTESIAN_POINT('Ctrl Pts',(0.493357799610229,-1.15634062715414,
0.9));
#13868=CARTESIAN_POINT('Ctrl Pts',(0.493357799610229,-1.15634062715414,
0.9));
#13869=CARTESIAN_POINT('Ctrl Pts',(0.495527690583772,-1.1541706728313,0.941427869885423));
#13870=CARTESIAN_POINT('Ctrl Pts',(0.497697580259374,-1.15200071970906,
0.982855739897088));
#13871=CARTESIAN_POINT('Ctrl Pts',(0.499867468632967,-1.14983076779109,
1.02428361003538));
#13872=CARTESIAN_POINT('Ctrl Pts',(12.8530083952718,-1.68438482323521,0.896653232994753));
#13873=CARTESIAN_POINT('Ctrl Pts',(12.8507727877026,-1.68214219351771,0.939311166602882));
#13874=CARTESIAN_POINT('Ctrl Pts',(12.8485371801548,-1.67989955599965,0.98196909980204));
#13875=CARTESIAN_POINT('Ctrl Pts',(12.8463015726285,-1.67765691065502,1.02462703259086));
#13876=CARTESIAN_POINT('Ctrl Pts',(12.852942348552,-1.70842230260233,0.897913479482771));
#13877=CARTESIAN_POINT('Ctrl Pts',(12.8507067417858,-1.70618025058462,0.940571446443912));
#13878=CARTESIAN_POINT('Ctrl Pts',(12.8484711274102,-1.70393818829512,0.983229412467123));
#13879=CARTESIAN_POINT('Ctrl Pts',(12.8462355206888,-1.70169612184244,1.02588737868196));
#13880=CARTESIAN_POINT('Ctrl Pts',(12.8409786353997,-1.75638702494578,0.899808108153313));
#13881=CARTESIAN_POINT('Ctrl Pts',(12.838742445636,-1.75414612041198,0.942466110756886));
#13882=CARTESIAN_POINT('Ctrl Pts',(12.8365062537503,-1.75190518941781,0.985124111849326));
#13883=CARTESIAN_POINT('Ctrl Pts',(12.8342700627828,-1.74966427281549,1.02778211378599));
#13884=CARTESIAN_POINT('Ctrl Pts',(12.7836010260412,-1.82153168011476,0.900225885582409));
#13885=CARTESIAN_POINT('Ctrl Pts',(12.7813622549889,-1.8192914414386,0.942883795866658));
#13886=CARTESIAN_POINT('Ctrl Pts',(12.7791234760524,-1.81705120036295,0.985541705643422));
#13887=CARTESIAN_POINT('Ctrl Pts',(12.7768846983302,-1.81481095080325,1.02819961506361));
#13888=CARTESIAN_POINT('Ctrl Pts',(12.7215544275214,-1.83731044697508,0.89780368869924));
#13889=CARTESIAN_POINT('Ctrl Pts',(12.7193134882941,-1.83506869652207,0.940461407834127));
#13890=CARTESIAN_POINT('Ctrl Pts',(12.7170725571902,-1.83282686943458,0.983119123314088));
#13891=CARTESIAN_POINT('Ctrl Pts',(12.7148316068824,-1.83058510462933,1.02577684117682));
#13892=CARTESIAN_POINT('Ctrl Pts',(12.6857439516282,-1.83320375805174,0.895711042712126));
#13893=CARTESIAN_POINT('Ctrl Pts',(12.6835023276506,-1.83096043753957,0.938368642889274));
#13894=CARTESIAN_POINT('Ctrl Pts',(12.6812606975378,-1.82871710814956,0.981026242308181));
#13895=CARTESIAN_POINT('Ctrl Pts',(12.6790190612712,-1.82647376985122,1.02368384096639));
#13896=CARTESIAN_POINT('',(12.685518570211,-1.83297820604925,0.9));
#13897=CARTESIAN_POINT('Ctrl Pts',(12.6790190612712,-1.82647376985122,1.02368384096639));
#13898=CARTESIAN_POINT('Ctrl Pts',(12.6811855699938,-1.8286419235626,0.982455894687418));
#13899=CARTESIAN_POINT('Ctrl Pts',(12.6833520729681,-1.83081006895277,0.941227947697881));
#13900=CARTESIAN_POINT('Ctrl Pts',(12.685518570211,-1.83297820604925,0.9));
#13901=CARTESIAN_POINT('Ctrl Pts',(12.685518570211,-1.83297820604925,0.9));
#13902=CARTESIAN_POINT('Ctrl Pts',(12.6962007718831,-1.83423224573831,0.900000000027109));
#13903=CARTESIAN_POINT('Ctrl Pts',(12.7069522081469,-1.8342814865544,0.899996797888993));
#13904=CARTESIAN_POINT('Ctrl Pts',(12.7175986228217,-1.83320546389923,0.899994443686255));
#13905=CARTESIAN_POINT('Ctrl Pts',(12.7263221437181,-1.83232378622612,0.899992514685985));
#13906=CARTESIAN_POINT('Ctrl Pts',(12.7349759538105,-1.83068541925521,0.899991134073322));
#13907=CARTESIAN_POINT('Ctrl Pts',(12.7434612806603,-1.82830833949467,0.899991022249493));
#13908=CARTESIAN_POINT('Ctrl Pts',(12.7538268490808,-1.82540452879472,0.899990885646912));
#13909=CARTESIAN_POINT('Ctrl Pts',(12.7638319405548,-1.82143037312377,0.899992779825431));
#13910=CARTESIAN_POINT('Ctrl Pts',(12.7733027638617,-1.81644210162737,0.899994914291513));
#13911=CARTESIAN_POINT('Ctrl Pts',(12.7785122133597,-1.81369829070399,0.899996088359796));
#13912=CARTESIAN_POINT('Ctrl Pts',(12.7835598637901,-1.81064675361041,0.899997279965736));
#13913=CARTESIAN_POINT('Ctrl Pts',(12.7884138119185,-1.80729078554336,0.899997716205233));
#13914=CARTESIAN_POINT('Ctrl Pts',(12.7907292666901,-1.80568990476168,0.899997924302393));
#13915=CARTESIAN_POINT('Ctrl Pts',(12.7930005978609,-1.80401968744988,0.8999979548189));
#13916=CARTESIAN_POINT('Ctrl Pts',(12.7952253950699,-1.80228259226775,0.89999788947913));
#13917=CARTESIAN_POINT('Ctrl Pts',(12.8036908359575,-1.7956728767752,0.899997640858734));
#13918=CARTESIAN_POINT('Ctrl Pts',(12.8113954895597,-1.78816822909976,0.899996334032805));
#13919=CARTESIAN_POINT('Ctrl Pts',(12.818232559256,-1.77993499666286,0.899996088064289));
#13920=CARTESIAN_POINT('Ctrl Pts',(12.8237887404903,-1.77324421631459,0.899995888176659));
#13921=CARTESIAN_POINT('Ctrl Pts',(12.8287718252447,-1.76607091125846,0.899996310183797));
#13922=CARTESIAN_POINT('Ctrl Pts',(12.8331051219922,-1.75848815553817,0.899996624147351));
#13923=CARTESIAN_POINT('Ctrl Pts',(12.8340140186356,-1.75689769413573,0.899996690000312));
#13924=CARTESIAN_POINT('Ctrl Pts',(12.8348928881302,-1.75529157361675,0.899996744625968));
#13925=CARTESIAN_POINT('Ctrl Pts',(12.8357411680586,-1.75367056321155,0.89999677208873));
#13926=CARTESIAN_POINT('Ctrl Pts',(12.8409005734958,-1.74381125896804,0.89999693912265));
#13927=CARTESIAN_POINT('Ctrl Pts',(12.8449329422938,-1.7334030651393,0.899996442311536));
#13928=CARTESIAN_POINT('Ctrl Pts',(12.8477914282597,-1.72264121193733,0.899997037599541));
#13929=CARTESIAN_POINT('Ctrl Pts',(12.850541038206,-1.71228926375309,0.899997610213799));
#13930=CARTESIAN_POINT('Ctrl Pts',(12.8521849869391,-1.70168212150629,0.899999138466857));
#13931=CARTESIAN_POINT('Ctrl Pts',(12.8526768248801,-1.69099162083728,0.899999779783946));
#13932=CARTESIAN_POINT('Ctrl Pts',(12.8527806949164,-1.68873392048611,0.899999915222113));
#13933=CARTESIAN_POINT('Ctrl Pts',(12.8528329986625,-1.68647247255235,0.90000000000128));
#13934=CARTESIAN_POINT('Ctrl Pts',(12.8528329986453,-1.6842088756636,0.9));
#13935=CARTESIAN_POINT('Origin',(6.88173176806555,0.,0.9));
#13936=CARTESIAN_POINT('Ctrl Pts',(12.685518570211,-1.83297820604925,0.9));
#13937=CARTESIAN_POINT('Ctrl Pts',(8.62146498001073,-1.3558778793304,0.9));
#13938=CARTESIAN_POINT('Ctrl Pts',(4.55741138981048,-1.2538870134557,0.9));
#13939=CARTESIAN_POINT('Ctrl Pts',(0.493357799610228,-1.15634062715414,
0.9));
#13940=CARTESIAN_POINT('Ctrl Pts',(12.685518570211,-1.83297820604925,0.9));
#13941=CARTESIAN_POINT('Ctrl Pts',(12.6834055233574,-1.83080706336992,0.941427870232769));
#13942=CARTESIAN_POINT('Ctrl Pts',(12.6812924765039,-1.8286359206906,0.982855740465538));
#13943=CARTESIAN_POINT('Ctrl Pts',(12.6791794296503,-1.82646477801127,1.02428361069831));
#13944=CARTESIAN_POINT('Ctrl Pts',(8.62146498001072,-1.3558778793304,0.9));
#13945=CARTESIAN_POINT('Ctrl Pts',(8.62076307594679,-1.35370673665108,0.941427870232769));
#13946=CARTESIAN_POINT('Ctrl Pts',(8.62006117188285,-1.35153559397175,0.982855740465538));
#13947=CARTESIAN_POINT('Ctrl Pts',(8.61935926781891,-1.34936445129242,1.02428361069831));
#13948=CARTESIAN_POINT('Ctrl Pts',(4.55741138981048,-1.2538870134557,0.9));
#13949=CARTESIAN_POINT('Ctrl Pts',(4.55812062853616,-1.25171587077637,0.941427870232769));
#13950=CARTESIAN_POINT('Ctrl Pts',(4.55882986726185,-1.24954472809705,0.982855740465538));
#13951=CARTESIAN_POINT('Ctrl Pts',(4.55953910598754,-1.24737358541772,1.02428361069831));
#13952=CARTESIAN_POINT('Ctrl Pts',(0.493357799610228,-1.15634062715414,
0.9));
#13953=CARTESIAN_POINT('Ctrl Pts',(0.495478181125536,-1.15416948447481,
0.941427870232769));
#13954=CARTESIAN_POINT('Ctrl Pts',(0.497598562640844,-1.15199834179549,
0.982855740465538));
#13955=CARTESIAN_POINT('Ctrl Pts',(0.499718944156152,-1.14982719911616,
1.02428361069831));
#19073=UNCERTAINTY_MEASURE_WITH_UNIT(LENGTH_MEASURE(0.001),#19091,
'DISTANCE_ACCURACY_VALUE',
'Maximum model space distance between geometric entities at asserted c
onnectivities');
#19077=UNCERTAINTY_MEASURE_WITH_UNIT(LENGTH_MEASURE(0.001),#19091,
'DISTANCE_ACCURACY_VALUE',
'Maximum model space distance between geometric entities at asserted c
onnectivities');
#19086=(
GEOMETRIC_REPRESENTATION_CONTEXT(3)
GLOBAL_UNCERTAINTY_ASSIGNED_CONTEXT((#19073))
GLOBAL_UNIT_ASSIGNED_CONTEXT((#19091,#19093,#19094))
REPRESENTATION_CONTEXT('','3D')
);
#19090=(
GEOMETRIC_REPRESENTATION_CONTEXT(3)
GLOBAL_UNCERTAINTY_ASSIGNED_CONTEXT((#19077))
GLOBAL_UNIT_ASSIGNED_CONTEXT((#19091,#19093,#19094))
REPRESENTATION_CONTEXT('','3D')
);
#19091=(
LENGTH_UNIT()
NAMED_UNIT(*)
SI_UNIT(.CENTI.,.METRE.)
);
#19093=(
NAMED_UNIT(*)
PLANE_ANGLE_UNIT()
SI_UNIT($,.RADIAN.)
);
#19094=(
NAMED_UNIT(*)
SI_UNIT($,.STERADIAN.)
SOLID_ANGLE_UNIT()
);
#19103=SHAPE_DEFINITION_REPRESENTATION(#19115,#19143);
#19115=PRODUCT_DEFINITION_SHAPE('',$,#19156);
#19143=SHAPE_REPRESENTATION('',(#7251),#19086);
#19147=PRODUCT_DEFINITION_CONTEXT('part definition',#19185,'design');
#19156=PRODUCT_DEFINITION('2026-11-10-05-09-19-263','Soft grip layer',#19168,
#19147);
#19168=PRODUCT_DEFINITION_FORMATION('',$,#19195);
#19185=APPLICATION_CONTEXT(
'Core Data for Automotive Mechanical Design Process');
#19186=PRODUCT_CONTEXT('part definition',#19185,'mechanical');
#19195=PRODUCT('2026-11-10-05-09-19-263','Soft grip layer',$,(#19186));
#19204=PRESENTATION_STYLE_ASSIGNMENT((#19212));
#19212=SURFACE_STYLE_USAGE(.BOTH.,#19220);
#19220=SURFACE_SIDE_STYLE('',(#19228));
#19228=SURFACE_STYLE_FILL_AREA(#19236);
#19236=FILL_AREA_STYLE('Sky blue soft grip',(#19244));
#19244=FILL_AREA_STYLE_COLOUR('Sky blue soft grip',#19252);
#19252=COLOUR_RGB('Sky blue soft grip',0.27843137254902,0.309803921568627,
0.352941176470588);
ENDSEC;
END-ISO-10303-21;
